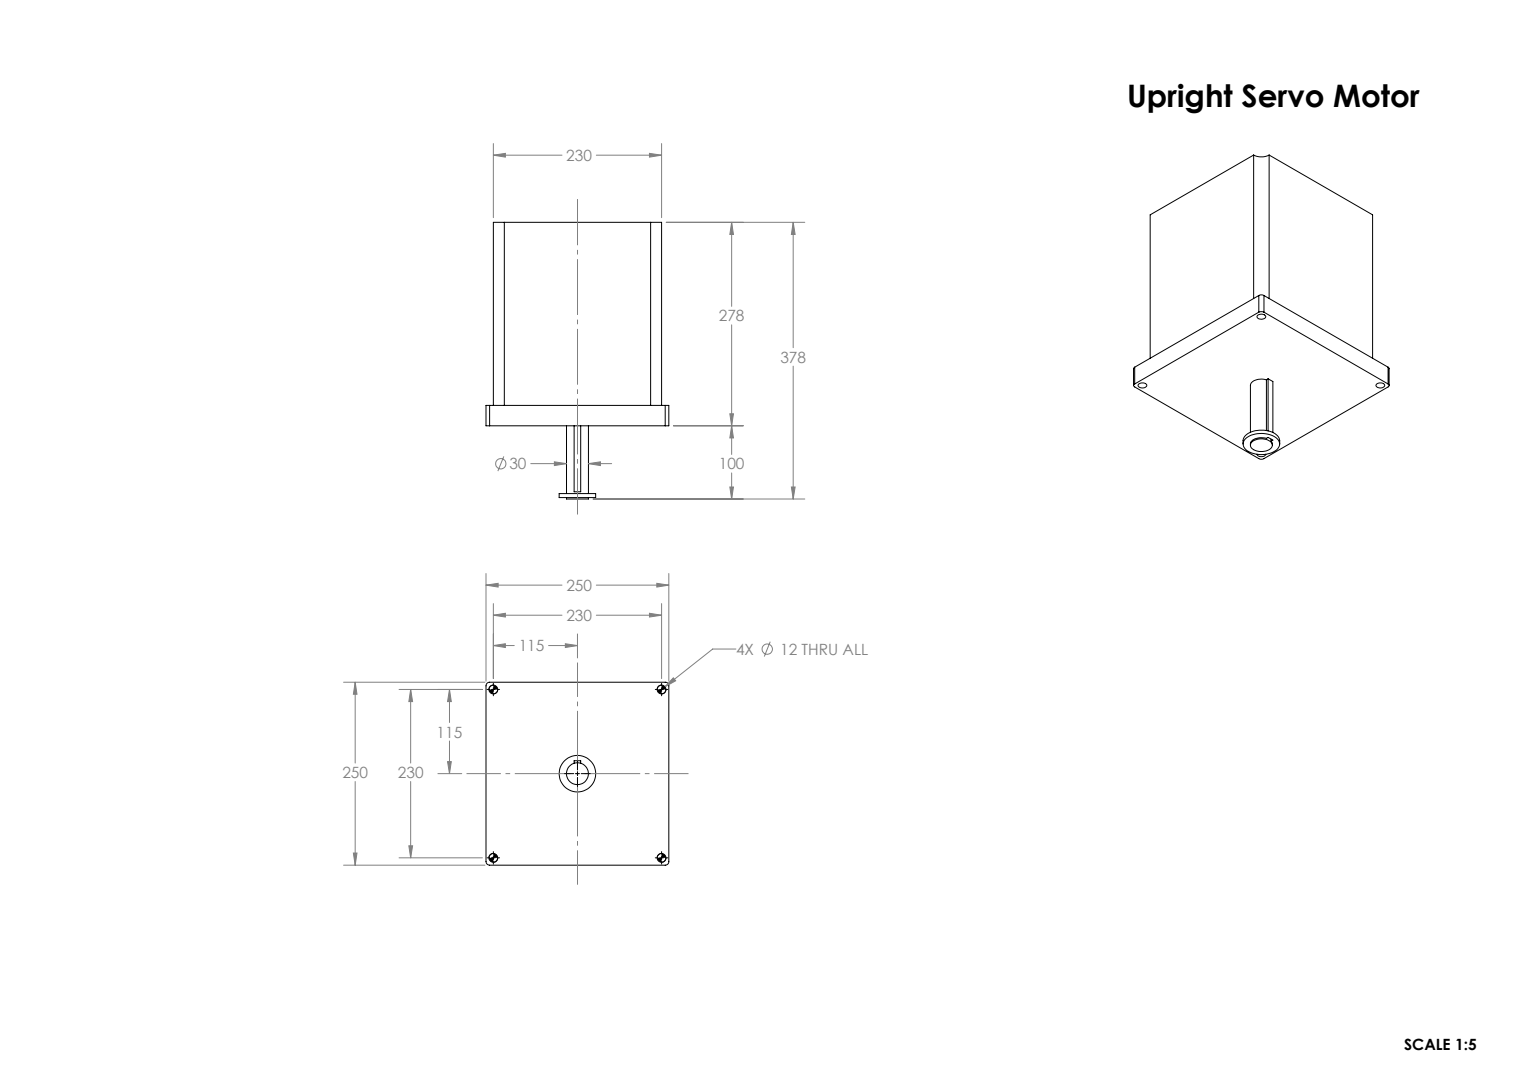
ISO-10303-21;
HEADER;
FILE_DESCRIPTION (('STEP AP214'),
    '1' );
FILE_NAME ('Upright servo motor.step',
    '2026-10-28T15:55:38',
    ( '' ),
    ( '' ),
    'SwSTEP 2.0',
    'SolidWorks 2025',
    '' );
FILE_SCHEMA (( 'AUTOMOTIVE_DESIGN' ));
ENDSEC;

DATA;
#1=CARTESIAN_POINT ( 'NONE',  ( -125.0000000000000000, -125.0000000000000000, 0.000000000000000000 ) ) ;
#8=CARTESIAN_POINT ( 'NONE',  ( 120.9999999999999005, 115.0000000000000000, -28.00000000000002487 ) ) ;
#18=ORIENTED_EDGE ( 'NONE', *, *, #6588, .T. ) ;
#27=CARTESIAN_POINT ( 'NONE',  ( -120.0000000000000000, 125.0000000000000000, -28.00000000000002487 ) ) ;
#29=ORIENTED_EDGE ( 'NONE', *, *, #180, .F. ) ;
#40=ADVANCED_FACE ( 'NONE', ( #3535 ), #4054, .T. ) ;
#42=ADVANCED_FACE ( 'NONE', ( #6164, #8163 ), #4942, .F. ) ;
#56=LINE ( 'NONE', #2567, #4947 ) ;
#61=EDGE_LOOP ( 'NONE', ( #697, #3265, #3475, #7513, #3300, #8064, #2980, #925, #7599, #4514 ) ) ;
#65=CARTESIAN_POINT ( 'NONE',  ( 120.0000000000000000, 125.0000000000000000, -28.00000000000002487 ) ) ;
#70=DIRECTION ( 'NONE',  ( 0.000000000000000000, 0.000000000000000000, -1.000000000000000000 ) ) ;
#72=ADVANCED_FACE ( 'NONE', ( #4004 ), #7908, .T. ) ;
#79=AXIS2_PLACEMENT_3D ( 'NONE', #2314, #7459, #4304 ) ;
#83=DIRECTION ( 'NONE',  ( -0.000000000000000000, -1.000000000000000000, 0.000000000000000000 ) ) ;
#105=CIRCLE ( 'NONE', #5900, 5.000000000000004441 ) ;
#108=VECTOR ( 'NONE', #4963, 1000.000000000000000 ) ;
#116=ORIENTED_EDGE ( 'NONE', *, *, #2238, .T. ) ;
#122=DIRECTION ( 'NONE',  ( 0.000000000000000000, 0.000000000000000000, -1.000000000000000000 ) ) ;
#141=LINE ( 'NONE', #5340, #3208 ) ;
#159=CARTESIAN_POINT ( 'NONE',  ( -114.9999999999999147, 115.0000000000000000, 8.205133554287239938E-16 ) ) ;
#173=DIRECTION ( 'NONE',  ( -1.000000000000000000, 0.000000000000000000, 0.000000000000000000 ) ) ;
#175=AXIS2_PLACEMENT_3D ( 'NONE', #7870, #4041, #5363 ) ;
#177=ADVANCED_FACE ( 'NONE', ( #1614 ), #1876, .F. ) ;
#179=VERTEX_POINT ( 'NONE', #7618 ) ;
#180=EDGE_CURVE ( 'NONE', #860, #2097, #1404, .T. ) ;
#181=FACE_OUTER_BOUND ( 'NONE', #3614, .T. ) ;
#183=CARTESIAN_POINT ( 'NONE',  ( -15.00000000000000000, 1.836970198721029589E-15, -120.5000000000000284 ) ) ;
#185=VECTOR ( 'NONE', #4186, 1000.000000000000000 ) ;
#190=EDGE_CURVE ( 'NONE', #8098, #1436, #474, .T. ) ;
#196=DIRECTION ( 'NONE',  ( -1.000000000000000000, 0.000000000000000000, 0.000000000000000000 ) ) ;
#198=EDGE_CURVE ( 'NONE', #5389, #4917, #4249, .T. ) ;
#207=ORIENTED_EDGE ( 'NONE', *, *, #1868, .F. ) ;
#208=DIRECTION ( 'NONE',  ( -0.000000000000000000, 0.000000000000000000, 1.000000000000000000 ) ) ;
#217=CARTESIAN_POINT ( 'NONE',  ( 17.61817604250836311, 0.000000000000000000, -28.00000000000002487 ) ) ;
#229=VECTOR ( 'NONE', #850, 1000.000000000000000 ) ;
#232=ORIENTED_EDGE ( 'NONE', *, *, #4651, .F. ) ;
#243=CIRCLE ( 'NONE', #6316, 15.00000000000001421 ) ;
#244=CIRCLE ( 'NONE', #3336, 5.999999999999991118 ) ;
#254=ORIENTED_EDGE ( 'NONE', *, *, #2828, .T. ) ;
#261=DIRECTION ( 'NONE',  ( -0.000000000000000000, -0.000000000000000000, -1.000000000000000000 ) ) ;
#271=CARTESIAN_POINT ( 'NONE',  ( 0.000000000000000000, -4.500000000000000000, -118.0000000000000284 ) ) ;
#286=EDGE_CURVE ( 'NONE', #441, #1522, #6503, .T. ) ;
#295=EDGE_CURVE ( 'NONE', #2535, #179, #3684, .T. ) ;
#300=CARTESIAN_POINT ( 'NONE',  ( -114.9999999999999147, 115.0000000000000000, 0.000000000000000000 ) ) ;
#304=DIRECTION ( 'NONE',  ( -0.000000000000000000, -0.000000000000000000, 1.000000000000000000 ) ) ;
#306=VERTEX_POINT ( 'NONE', #4470 ) ;
#308=EDGE_CURVE ( 'NONE', #902, #5541, #1677, .T. ) ;
#310=CLOSED_SHELL ( 'NONE', ( #3649, #1499, #7471, #6289, #6383, #2621, #654, #8259, #5840, #40, #7066, #4000, #7991, #7178, #2940, #72, #5941, #5722, #5455, #6114, #6194, #3420, #920, #177, #2590, #2030, #4073, #5503, #4001, #3296, #1919, #610, #4469, #5040, #3468, #42, #666, #5099, #4929, #6667, #3666 ) ) ;
#315=CARTESIAN_POINT ( 'NONE',  ( 0.000000000000000000, 0.000000000000000000, -128.0000000000000284 ) ) ;
#326=VERTEX_POINT ( 'NONE', #1488 ) ;
#331=LINE ( 'NONE', #1063, #1617 ) ;
#342=( NAMED_UNIT ( * ) SI_UNIT ( $, .STERADIAN. ) SOLID_ANGLE_UNIT ( ) );
#347=DIRECTION ( 'NONE',  ( -1.000000000000000000, 0.000000000000000000, -0.000000000000000000 ) ) ;
#350=AXIS2_PLACEMENT_3D ( 'NONE', #7544, #3683, #6944 ) ;
#352=DIRECTION ( 'NONE',  ( 1.000000000000000000, 0.000000000000000000, 0.000000000000000000 ) ) ;
#370=CARTESIAN_POINT ( 'NONE',  ( 0.000000000000000000, 0.000000000000000000, -120.5000000000000284 ) ) ;
#371=AXIS2_PLACEMENT_3D ( 'NONE', #2070, #6035, #7190 ) ;
#377=AXIS2_PLACEMENT_3D ( 'NONE', #5650, #8275, #3063 ) ;
#380=DIRECTION ( 'NONE',  ( -1.000000000000000000, 0.000000000000000000, 0.000000000000000000 ) ) ;
#381=VERTEX_POINT ( 'NONE', #27 ) ;
#383=AXIS2_PLACEMENT_3D ( 'NONE', #486, #7032, #3735 ) ;
#407=ORIENTED_EDGE ( 'NONE', *, *, #3693, .F. ) ;
#411=LINE ( 'NONE', #3703, #3911 ) ;
#415=FACE_OUTER_BOUND ( 'NONE', #707, .T. ) ;
#428=LINE ( 'NONE', #8161, #3975 ) ;
#430=CARTESIAN_POINT ( 'NONE',  ( 114.9999999999999147, 115.0000000000000000, 0.000000000000000000 ) ) ;
#433=EDGE_LOOP ( 'NONE', ( #2336, #6110, #4542, #3751 ) ) ;
#441=VERTEX_POINT ( 'NONE', #3239 ) ;
#450=DIRECTION ( 'NONE',  ( -1.000000000000000000, 0.000000000000000000, 0.000000000000000000 ) ) ;
#455=PLANE ( 'NONE',  #2955 ) ;
#465=CARTESIAN_POINT ( 'NONE',  ( -120.0000000000000000, -125.0000000000000000, 0.000000000000000000 ) ) ;
#471=VERTEX_POINT ( 'NONE', #3527 ) ;
#474=LINE ( 'NONE', #5587, #3002 ) ;
#475=FACE_OUTER_BOUND ( 'NONE', #6736, .T. ) ;
#486=CARTESIAN_POINT ( 'NONE',  ( -114.9999999999999147, -115.0000000000000000, 250.0000000000000000 ) ) ;
#493=DIRECTION ( 'NONE',  ( -0.000000000000000000, -0.000000000000000000, 1.000000000000000000 ) ) ;
#506=CARTESIAN_POINT ( 'NONE',  ( 17.61817604250836311, 0.000000000000000000, -128.0000120000000265 ) ) ;
#515=ORIENTED_EDGE ( 'NONE', *, *, #1831, .T. ) ;
#534=CIRCLE ( 'NONE', #1490, 5.000000000000004441 ) ;
#535=CARTESIAN_POINT ( 'NONE',  ( 0.000000000000000000, 0.000000000000000000, -128.0000000000000284 ) ) ;
#536=AXIS2_PLACEMENT_3D ( 'NONE', #6714, #5911, #8024 ) ;
#538=FACE_OUTER_BOUND ( 'NONE', #2255, .T. ) ;
#546=ORIENTED_EDGE ( 'NONE', *, *, #4676, .T. ) ;
#548=CARTESIAN_POINT ( 'NONE',  ( -125.0000000000000000, 125.0000000000000000, -28.00000000000002487 ) ) ;
#552=ORIENTED_EDGE ( 'NONE', *, *, #875, .F. ) ;
#559=ORIENTED_EDGE ( 'NONE', *, *, #4204, .F. ) ;
#565=DIRECTION ( 'NONE',  ( -1.000000000000000000, 0.000000000000000000, -0.000000000000000000 ) ) ;
#566=DIRECTION ( 'NONE',  ( -0.000000000000000000, -0.000000000000000000, 1.000000000000000000 ) ) ;
#570=EDGE_CURVE ( 'NONE', #6321, #3267, #1593, .T. ) ;
#578=FACE_OUTER_BOUND ( 'NONE', #61, .T. ) ;
#581=EDGE_CURVE ( 'NONE', #7933, #4405, #6106, .T. ) ;
#583=AXIS2_PLACEMENT_3D ( 'NONE', #4746, #5934, #7328 ) ;
#589=LINE ( 'NONE', #629, #1204 ) ;
#593=EDGE_LOOP ( 'NONE', ( #552, #7812 ) ) ;
#607=CIRCLE ( 'NONE', #7489, 5.999999999999991118 ) ;
#610=ADVANCED_FACE ( 'NONE', ( #5041 ), #4306, .T. ) ;
#612=EDGE_LOOP ( 'NONE', ( #6446, #1124, #2582, #4474, #7041 ) ) ;
#615=EDGE_CURVE ( 'NONE', #4158, #3739, #1807, .T. ) ;
#620=DIRECTION ( 'NONE',  ( 1.000000000000000000, -0.000000000000000000, 0.000000000000000000 ) ) ;
#629=CARTESIAN_POINT ( 'NONE',  ( -120.0000000000000000, -125.0000000000000000, -28.00000000000002487 ) ) ;
#633=VECTOR ( 'NONE', #208, 1000.000000000000000 ) ;
#644=LINE ( 'NONE', #2550, #3740 ) ;
#645=CARTESIAN_POINT ( 'NONE',  ( 114.9999999999999147, 115.0000000000000000, 250.0000000000000000 ) ) ;
#654=ADVANCED_FACE ( 'NONE', ( #5169 ), #7069, .F. ) ;
#659=DIRECTION ( 'NONE',  ( -1.000000000000000000, 0.000000000000000000, 0.000000000000000000 ) ) ;
#666=ADVANCED_FACE ( 'NONE', ( #5376 ), #6607, .T. ) ;
#668=ORIENTED_EDGE ( 'NONE', *, *, #4872, .F. ) ;
#672=EDGE_LOOP ( 'NONE', ( #3276, #4594, #7730, #8070 ) ) ;
#687=ORIENTED_EDGE ( 'NONE', *, *, #3635, .T. ) ;
#697=ORIENTED_EDGE ( 'NONE', *, *, #8210, .F. ) ;
#698=VERTEX_POINT ( 'NONE', #4611 ) ;
#703=LINE ( 'NONE', #5265, #4111 ) ;
#705=EDGE_LOOP ( 'NONE', ( #4300, #4268, #4984, #5088 ) ) ;
#706=MANIFOLD_SOLID_BREP ( 'Cut-Extrude1', #310 ) ;
#707=EDGE_LOOP ( 'NONE', ( #6265, #1176, #18, #8160, #1408, #795, #3196, #6738 ) ) ;
#720=CARTESIAN_POINT ( 'NONE',  ( 17.61817604250836311, 0.000000000000000000, -118.0000000000000284 ) ) ;
#733=DIRECTION ( 'NONE',  ( 0.000000000000000000, 0.000000000000000000, -1.000000000000000000 ) ) ;
#735=EDGE_CURVE ( 'NONE', #3015, #3602, #6056, .T. ) ;
#740=EDGE_CURVE ( 'NONE', #2575, #6246, #8045, .T. ) ;
#741=LINE ( 'NONE', #2603, #1864 ) ;
#744=LINE ( 'NONE', #906, #4238 ) ;
#748=ORIENTED_EDGE ( 'NONE', *, *, #2964, .F. ) ;
#751=CARTESIAN_POINT ( 'NONE',  ( -15.00000000000000000, 1.836970198721029589E-15, -128.0000000000000284 ) ) ;
#753=AXIS2_PLACEMENT_3D ( 'NONE', #5334, #785, #7918 ) ;
#755=EDGE_LOOP ( 'NONE', ( #6173, #4215, #4913, #5960 ) ) ;
#763=DIRECTION ( 'NONE',  ( -1.000000000000000000, 0.000000000000000000, 0.000000000000000000 ) ) ;
#766=LINE ( 'NONE', #1, #7092 ) ;
#776=PLANE ( 'NONE',  #6139 ) ;
#785=DIRECTION ( 'NONE',  ( 0.000000000000000000, 0.000000000000000000, 1.000000000000000000 ) ) ;
#786=CARTESIAN_POINT ( 'NONE',  ( 114.9999999999999147, 115.0000000000000000, 8.205133554287239938E-16 ) ) ;
#789=ORIENTED_EDGE ( 'NONE', *, *, #1988, .T. ) ;
#795=ORIENTED_EDGE ( 'NONE', *, *, #6434, .F. ) ;
#797=DIRECTION ( 'NONE',  ( 1.000000000000000000, 0.000000000000000000, 0.000000000000000000 ) ) ;
#802=CIRCLE ( 'NONE', #2559, 15.00000000000000178 ) ;
#805=VERTEX_POINT ( 'NONE', #4712 ) ;
#823=CARTESIAN_POINT ( 'NONE',  ( 0.000000000000000000, 0.000000000000000000, -128.0000000000000284 ) ) ;
#827=CARTESIAN_POINT ( 'NONE',  ( -15.00000000000000000, 1.836970198721029589E-15, -126.0000000000000284 ) ) ;
#831=DIRECTION ( 'NONE',  ( 1.000000000000000000, 0.000000000000000000, 0.000000000000000000 ) ) ;
#838=CARTESIAN_POINT ( 'NONE',  ( 0.000000000000000000, 4.500000000000000000, -126.0000000000000284 ) ) ;
#850=DIRECTION ( 'NONE',  ( -0.000000000000000000, -0.000000000000000000, 1.000000000000000000 ) ) ;
#857=CARTESIAN_POINT ( 'NONE',  ( 17.61817604250836311, 0.000000000000000000, -126.0000000000000284 ) ) ;
#859=EDGE_LOOP ( 'NONE', ( #1022, #5933, #4897, #7019 ) ) ;
#860=VERTEX_POINT ( 'NONE', #1420 ) ;
#869=DIRECTION ( 'NONE',  ( 1.000000000000000000, 0.000000000000000000, 0.000000000000000000 ) ) ;
#872=DIRECTION ( 'NONE',  ( -1.000000000000000000, 0.000000000000000000, 0.000000000000000000 ) ) ;
#875=EDGE_CURVE ( 'NONE', #5541, #902, #607, .T. ) ;
#897=CIRCLE ( 'NONE', #5065, 15.00000000000000000 ) ;
#900=VERTEX_POINT ( 'NONE', #1546 ) ;
#901=CIRCLE ( 'NONE', #2392, 5.999999999999991118 ) ;
#902=VERTEX_POINT ( 'NONE', #2874 ) ;
#906=CARTESIAN_POINT ( 'NONE',  ( -0.000000000000000000, -115.0000000000000000, 0.000000000000000000 ) ) ;
#911=VECTOR ( 'NONE', #1701, 1000.000000000000000 ) ;
#913=CIRCLE ( 'NONE', #5356, 15.00000000000000000 ) ;
#920=ADVANCED_FACE ( 'NONE', ( #4178 ), #7961, .T. ) ;
#925=ORIENTED_EDGE ( 'NONE', *, *, #2471, .F. ) ;
#926=CARTESIAN_POINT ( 'NONE',  ( -125.0000000000000000, -120.0000000000000000, 0.000000000000000000 ) ) ;
#934=CARTESIAN_POINT ( 'NONE',  ( -15.00000000000000000, 1.836970198721029589E-15, -128.0000000000000284 ) ) ;
#959=CARTESIAN_POINT ( 'NONE',  ( 125.0000000000000000, -120.0000000000000000, 0.000000000000000000 ) ) ;
#960=ORIENTED_EDGE ( 'NONE', *, *, #2835, .F. ) ;
#973=EDGE_CURVE ( 'NONE', #860, #2535, #428, .T. ) ;
#974=DIRECTION ( 'NONE',  ( -1.000000000000000000, 0.000000000000000000, 0.000000000000000000 ) ) ;
#991=EDGE_CURVE ( 'NONE', #1826, #2040, #4912, .T. ) ;
#998=DIRECTION ( 'NONE',  ( -0.000000000000000000, -0.000000000000000000, 1.000000000000000000 ) ) ;
#1006=VECTOR ( 'NONE', #4028, 1000.000000000000000 ) ;
#1010=VERTEX_POINT ( 'NONE', #7054 ) ;
#1011=DIRECTION ( 'NONE',  ( 1.000000000000000000, 0.000000000000000000, 0.000000000000000000 ) ) ;
#1013=EDGE_LOOP ( 'NONE', ( #559, #6984, #2873, #7573 ) ) ;
#1018=ORIENTED_EDGE ( 'NONE', *, *, #3827, .T. ) ;
#1022=ORIENTED_EDGE ( 'NONE', *, *, #5036, .F. ) ;
#1026=EDGE_CURVE ( 'NONE', #4868, #3146, #766, .T. ) ;
#1036=FACE_BOUND ( 'NONE', #3299, .T. ) ;
#1039=CIRCLE ( 'NONE', #8188, 15.00000000000000000 ) ;
#1040=CARTESIAN_POINT ( 'NONE',  ( 120.9999999999999005, 115.0000000000000000, 0.000000000000000000 ) ) ;
#1046=EDGE_CURVE ( 'NONE', #1156, #5510, #1993, .T. ) ;
#1052=DIRECTION ( 'NONE',  ( 0.000000000000000000, 0.000000000000000000, -1.000000000000000000 ) ) ;
#1055=ORIENTED_EDGE ( 'NONE', *, *, #2141, .T. ) ;
#1056=CIRCLE ( 'NONE', #2670, 14.99999999999998579 ) ;
#1057=ORIENTED_EDGE ( 'NONE', *, *, #4872, .T. ) ;
#1063=CARTESIAN_POINT ( 'NONE',  ( 114.9999999999999147, -100.0000000000000000, 250.0000000000000000 ) ) ;
#1092=CARTESIAN_POINT ( 'NONE',  ( 114.9999999999999147, 99.99999999999998579, 250.0000000000000000 ) ) ;
#1100=EDGE_LOOP ( 'NONE', ( #2705, #116, #7783, #4128 ) ) ;
#1104=LINE ( 'NONE', #3664, #3805 ) ;
#1108=ORIENTED_EDGE ( 'NONE', *, *, #1831, .F. ) ;
#1114=ORIENTED_EDGE ( 'NONE', *, *, #740, .F. ) ;
#1116=DIRECTION ( 'NONE',  ( -0.000000000000000000, -0.000000000000000000, -1.000000000000000000 ) ) ;
#1124=ORIENTED_EDGE ( 'NONE', *, *, #6601, .F. ) ;
#1128=FACE_BOUND ( 'NONE', #2832, .T. ) ;
#1135=EDGE_CURVE ( 'NONE', #5480, #5616, #901, .T. ) ;
#1139=LINE ( 'NONE', #6232, #5220 ) ;
#1151=CARTESIAN_POINT ( 'NONE',  ( 120.0000000000000000, 120.0000000000000000, 0.000000000000000000 ) ) ;
#1153=ORIENTED_EDGE ( 'NONE', *, *, #2768, .T. ) ;
#1156=VERTEX_POINT ( 'NONE', #7787 ) ;
#1170=DIRECTION ( 'NONE',  ( 0.000000000000000000, -0.000000000000000000, -1.000000000000000000 ) ) ;
#1174=DIRECTION ( 'NONE',  ( -0.000000000000000000, -0.000000000000000000, -1.000000000000000000 ) ) ;
#1176=ORIENTED_EDGE ( 'NONE', *, *, #7255, .T. ) ;
#1178=ORIENTED_EDGE ( 'NONE', *, *, #7163, .F. ) ;
#1193=EDGE_LOOP ( 'NONE', ( #3836, #2902 ) ) ;
#1196=CARTESIAN_POINT ( 'NONE',  ( 114.9999999999999147, -100.0000000000000000, 250.0000000000000000 ) ) ;
#1204=VECTOR ( 'NONE', #7735, 1000.000000000000000 ) ;
#1215=LINE ( 'NONE', #3138, #8195 ) ;
#1220=ORIENTED_EDGE ( 'NONE', *, *, #740, .T. ) ;
#1223=ORIENTED_EDGE ( 'NONE', *, *, #8210, .T. ) ;
#1224=DIRECTION ( 'NONE',  ( -0.000000000000000000, -0.000000000000000000, 1.000000000000000000 ) ) ;
#1230=ORIENTED_EDGE ( 'NONE', *, *, #5274, .T. ) ;
#1236=LINE ( 'NONE', #5104, #2277 ) ;
#1242=CARTESIAN_POINT ( 'NONE',  ( -114.9999999999999147, -115.0000000000000000, -28.00000000000002487 ) ) ;
#1246=DIRECTION ( 'NONE',  ( 1.000000000000000000, 0.000000000000000000, 0.000000000000000000 ) ) ;
#1258=PLANE ( 'NONE',  #5615 ) ;
#1259=AXIS2_PLACEMENT_3D ( 'NONE', #645, #5115, #2551 ) ;
#1264=DIRECTION ( 'NONE',  ( 1.000000000000000000, 0.000000000000000000, 0.000000000000000000 ) ) ;
#1273=EDGE_CURVE ( 'NONE', #2993, #326, #2375, .T. ) ;
#1278=DIRECTION ( 'NONE',  ( -0.000000000000000000, -0.000000000000000000, 1.000000000000000000 ) ) ;
#1285=EDGE_CURVE ( 'NONE', #2048, #805, #1104, .T. ) ;
#1291=FACE_OUTER_BOUND ( 'NONE', #6963, .T. ) ;
#1298=FACE_OUTER_BOUND ( 'NONE', #2580, .T. ) ;
#1299=AXIS2_PLACEMENT_3D ( 'NONE', #5884, #1507, #5927 ) ;
#1315=CIRCLE ( 'NONE', #79, 5.999999999999991118 ) ;
#1322=VECTOR ( 'NONE', #6685, 1000.000000000000000 ) ;
#1332=CARTESIAN_POINT ( 'NONE',  ( 108.9999999999999147, 115.0000000000000000, 8.205133554287239938E-16 ) ) ;
#1338=AXIS2_PLACEMENT_3D ( 'NONE', #7250, #6573, #797 ) ;
#1352=AXIS2_PLACEMENT_3D ( 'NONE', #2473, #566, #6940 ) ;
#1364=DIRECTION ( 'NONE',  ( -1.000000000000000000, 0.000000000000000000, 0.000000000000000000 ) ) ;
#1373=DIRECTION ( 'NONE',  ( -1.000000000000000000, 0.000000000000000000, 0.000000000000000000 ) ) ;
#1402=VERTEX_POINT ( 'NONE', #5132 ) ;
#1403=DIRECTION ( 'NONE',  ( 0.000000000000000000, 0.000000000000000000, 1.000000000000000000 ) ) ;
#1404=CIRCLE ( 'NONE', #2867, 5.999999999999991118 ) ;
#1408=ORIENTED_EDGE ( 'NONE', *, *, #7184, .F. ) ;
#1420=CARTESIAN_POINT ( 'NONE',  ( -120.9999999999999005, 115.0000000000000000, -28.00000000000002487 ) ) ;
#1436=VERTEX_POINT ( 'NONE', #2152 ) ;
#1439=EDGE_CURVE ( 'NONE', #3146, #2918, #7043, .T. ) ;
#1440=SHAPE_REPRESENTATION ( 'Upright servo motor', ( #1299 ), #7463 ) ;
#1446=VECTOR ( 'NONE', #1666, 1000.000000000000000 ) ;
#1457=CIRCLE ( 'NONE', #3320, 25.00000000000000000 ) ;
#1465=AXIS2_PLACEMENT_3D ( 'NONE', #1830, #7610, #3840 ) ;
#1468=ORIENTED_EDGE ( 'NONE', *, *, #7255, .F. ) ;
#1474=LINE ( 'NONE', #6445, #5413 ) ;
#1479=CARTESIAN_POINT ( 'NONE',  ( 108.9999999999999147, 115.0000000000000000, -28.00000000000002487 ) ) ;
#1488=CARTESIAN_POINT ( 'NONE',  ( -114.9999999999999147, 99.99999999999998579, 0.000000000000000000 ) ) ;
#1490=AXIS2_PLACEMENT_3D ( 'NONE', #6464, #733, #6414 ) ;
#1499=ADVANCED_FACE ( 'NONE', ( #6568 ), #3346, .F. ) ;
#1504=CARTESIAN_POINT ( 'NONE',  ( 0.000000000000000000, 0.000000000000000000, -118.0000000000000284 ) ) ;
#1507=DIRECTION ( 'NONE',  ( 0.000000000000000000, 0.000000000000000000, 1.000000000000000000 ) ) ;
#1510=ORIENTED_EDGE ( 'NONE', *, *, #2685, .F. ) ;
#1513=CARTESIAN_POINT ( 'NONE',  ( 114.9999999999999147, 115.0000000000000000, 250.0000000000000000 ) ) ;
#1521=CARTESIAN_POINT ( 'NONE',  ( 0.000000000000000000, 0.000000000000000000, -118.0000000000000284 ) ) ;
#1522=VERTEX_POINT ( 'NONE', #6085 ) ;
#1531=CYLINDRICAL_SURFACE ( 'NONE', #1465, 5.000000000000004441 ) ;
#1546=CARTESIAN_POINT ( 'NONE',  ( 108.9999999999999147, -115.0000000000000000, 8.205133554287239938E-16 ) ) ;
#1550=AXIS2_PLACEMENT_3D ( 'NONE', #7363, #4133, #173 ) ;
#1554=DIRECTION ( 'NONE',  ( -0.000000000000000000, -0.000000000000000000, 1.000000000000000000 ) ) ;
#1558=( NAMED_UNIT ( * ) PLANE_ANGLE_UNIT ( ) SI_UNIT ( $, .RADIAN. ) );
#1563=CARTESIAN_POINT ( 'NONE',  ( 0.000000000000000000, -115.0000000000000000, 250.0000000000000000 ) ) ;
#1573=PLANE ( 'NONE',  #536 ) ;
#1587=DIRECTION ( 'NONE',  ( 0.000000000000000000, 1.000000000000000000, 0.000000000000000000 ) ) ;
#1593=LINE ( 'NONE', #4103, #1006 ) ;
#1602=ORIENTED_EDGE ( 'NONE', *, *, #1646, .T. ) ;
#1606=ORIENTED_EDGE ( 'NONE', *, *, #3419, .F. ) ;
#1607=CARTESIAN_POINT ( 'NONE',  ( 0.000000000000000000, 0.000000000000000000, -28.00000000000002487 ) ) ;
#1610=CARTESIAN_POINT ( 'NONE',  ( -108.9999999999999147, 115.0000000000000000, -28.00000000000002487 ) ) ;
#1612=DIRECTION ( 'NONE',  ( -1.000000000000000000, 0.000000000000000000, 0.000000000000000000 ) ) ;
#1614=FACE_OUTER_BOUND ( 'NONE', #3031, .T. ) ;
#1617=VECTOR ( 'NONE', #3669, 1000.000000000000000 ) ;
#1618=VERTEX_POINT ( 'NONE', #2962 ) ;
#1642=CARTESIAN_POINT ( 'NONE',  ( 0.000000000000000000, 4.500000000000000000, -28.00000000000002487 ) ) ;
#1646=EDGE_CURVE ( 'NONE', #3602, #4182, #8060, .T. ) ;
#1659=CARTESIAN_POINT ( 'NONE',  ( -99.99999999999990052, 115.0000000000000000, 250.0000000000000000 ) ) ;
#1666=DIRECTION ( 'NONE',  ( -0.000000000000000000, -0.000000000000000000, -1.000000000000000000 ) ) ;
#1677=CIRCLE ( 'NONE', #8291, 5.999999999999991118 ) ;
#1680=VERTEX_POINT ( 'NONE', #4849 ) ;
#1701=DIRECTION ( 'NONE',  ( -0.000000000000000000, -0.000000000000000000, -1.000000000000000000 ) ) ;
#1712=PLANE ( 'NONE',  #6288 ) ;
#1714=ORIENTED_EDGE ( 'NONE', *, *, #3909, .F. ) ;
#1720=AXIS2_PLACEMENT_3D ( 'NONE', #4653, #6681, #4610 ) ;
#1725=DIRECTION ( 'NONE',  ( 0.000000000000000000, 0.000000000000000000, 1.000000000000000000 ) ) ;
#1728=EDGE_LOOP ( 'NONE', ( #232, #5693, #3645, #5839 ) ) ;
#1739=DIRECTION ( 'NONE',  ( -0.000000000000000000, -0.000000000000000000, 1.000000000000000000 ) ) ;
#1745=EDGE_CURVE ( 'NONE', #7187, #2575, #4891, .T. ) ;
#1764=FACE_BOUND ( 'NONE', #612, .T. ) ;
#1767=DIRECTION ( 'NONE',  ( -1.000000000000000000, 0.000000000000000000, 0.000000000000000000 ) ) ;
#1776=ORIENTED_EDGE ( 'NONE', *, *, #4676, .F. ) ;
#1787=VERTEX_POINT ( 'NONE', #3399 ) ;
#1788=ORIENTED_EDGE ( 'NONE', *, *, #1439, .T. ) ;
#1794=LINE ( 'NONE', #3627, #6152 ) ;
#1795=AXIS2_PLACEMENT_3D ( 'NONE', #3418, #3382, #872 ) ;
#1807=LINE ( 'NONE', #1040, #8016 ) ;
#1808=CARTESIAN_POINT ( 'NONE',  ( 0.000000000000000000, 115.0000000000000000, 250.0000000000000000 ) ) ;
#1814=AXIS2_PLACEMENT_3D ( 'NONE', #3162, #8332, #5070 ) ;
#1818=CARTESIAN_POINT ( 'NONE',  ( -120.9999999999999005, -115.0000000000000000, -28.00000000000002487 ) ) ;
#1826=VERTEX_POINT ( 'NONE', #2707 ) ;
#1828=MECHANICAL_DESIGN_GEOMETRIC_PRESENTATION_REPRESENTATION('',(#3014),#4768);
#1830=CARTESIAN_POINT ( 'NONE',  ( -120.0000000000000000, 120.0000000000000000, -28.00000000000002487 ) ) ;
#1831=EDGE_CURVE ( 'NONE', #900, #7564, #7396, .T. ) ;
#1843=CYLINDRICAL_SURFACE ( 'NONE', #2399, 5.999999999999991118 ) ;
#1845=LINE ( 'NONE', #8344, #3612 ) ;
#1855=UNCERTAINTY_MEASURE_WITH_UNIT (LENGTH_MEASURE( 1.000000000000000082E-05 ), #3540, 'distance_accuracy_value', 'NONE');
#1856=ORIENTED_EDGE ( 'NONE', *, *, #6275, .T. ) ;
#1859=EDGE_LOOP ( 'NONE', ( #789, #2881, #5851, #4229, #5350 ) ) ;
#1860=CARTESIAN_POINT ( 'NONE',  ( 0.000000000000000000, 4.500000000000000000, -118.0000000000000284 ) ) ;
#1864=VECTOR ( 'NONE', #5763, 1000.000000000000000 ) ;
#1868=EDGE_CURVE ( 'NONE', #5616, #5480, #4408, .T. ) ;
#1876=CYLINDRICAL_SURFACE ( 'NONE', #1814, 15.00000000000000000 ) ;
#1886=CARTESIAN_POINT ( 'NONE',  ( 0.000000000000000000, 0.000000000000000000, -126.0000000000000284 ) ) ;
#1891=ORIENTED_EDGE ( 'NONE', *, *, #7608, .F. ) ;
#1919=ADVANCED_FACE ( 'NONE', ( #2008 ), #5194, .T. ) ;
#1920=DIRECTION ( 'NONE',  ( 1.000000000000000000, 0.000000000000000000, 0.000000000000000000 ) ) ;
#1925=CARTESIAN_POINT ( 'NONE',  ( 17.61817604250836311, 4.500000000000000000, -120.5000000000000284 ) ) ;
#1928=DIRECTION ( 'NONE',  ( 1.000000000000000000, 0.000000000000000000, 0.000000000000000000 ) ) ;
#1937=DIRECTION ( 'NONE',  ( 0.000000000000000000, 1.000000000000000000, 0.000000000000000000 ) ) ;
#1938=EDGE_CURVE ( 'NONE', #5315, #1010, #2286, .T. ) ;
#1939=LINE ( 'NONE', #1808, #6729 ) ;
#1962=VERTEX_POINT ( 'NONE', #3358 ) ;
#1963=ORIENTED_EDGE ( 'NONE', *, *, #4837, .F. ) ;
#1978=ORIENTED_EDGE ( 'NONE', *, *, #1026, .F. ) ;
#1988=EDGE_CURVE ( 'NONE', #1680, #6868, #7261, .T. ) ;
#1990=EDGE_CURVE ( 'NONE', #4182, #4386, #8216, .T. ) ;
#1992=ORIENTED_EDGE ( 'NONE', *, *, #5607, .F. ) ;
#1993=CIRCLE ( 'NONE', #3040, 25.00000000000000000 ) ;
#2008=FACE_OUTER_BOUND ( 'NONE', #8041, .T. ) ;
#2016=DIRECTION ( 'NONE',  ( 1.000000000000000000, 0.000000000000000000, 0.000000000000000000 ) ) ;
#2019=VERTEX_POINT ( 'NONE', #3396 ) ;
#2029=FACE_OUTER_BOUND ( 'NONE', #6543, .T. ) ;
#2030=ADVANCED_FACE ( 'NONE', ( #415 ), #8104, .T. ) ;
#2040=VERTEX_POINT ( 'NONE', #8147 ) ;
#2044=VECTOR ( 'NONE', #3445, 1000.000000000000000 ) ;
#2048=VERTEX_POINT ( 'NONE', #6067 ) ;
#2050=VECTOR ( 'NONE', #7364, 1000.000000000000000 ) ;
#2055=DIRECTION ( 'NONE',  ( -1.000000000000000000, 0.000000000000000000, 0.000000000000000000 ) ) ;
#2058=DIRECTION ( 'NONE',  ( -0.000000000000000000, -0.000000000000000000, -1.000000000000000000 ) ) ;
#2070=CARTESIAN_POINT ( 'NONE',  ( 114.9999999999999147, -115.0000000000000000, 8.205133554287239938E-16 ) ) ;
#2097=VERTEX_POINT ( 'NONE', #1610 ) ;
#2098=AXIS2_PLACEMENT_3D ( 'NONE', #4174, #6763, #5459 ) ;
#2102=DIRECTION ( 'NONE',  ( -0.000000000000000000, -0.000000000000000000, 1.000000000000000000 ) ) ;
#2104=LINE ( 'NONE', #5410, #2044 ) ;
#2108=CARTESIAN_POINT ( 'NONE',  ( 0.000000000000000000, 0.000000000000000000, -118.0000000000000284 ) ) ;
#2119=ORIENTED_EDGE ( 'NONE', *, *, #2298, .T. ) ;
#2132=CARTESIAN_POINT ( 'NONE',  ( 0.000000000000000000, 0.000000000000000000, -28.00000000000002487 ) ) ;
#2137=FACE_OUTER_BOUND ( 'NONE', #8280, .T. ) ;
#2140=CYLINDRICAL_SURFACE ( 'NONE', #5625, 25.00000000000000000 ) ;
#2141=EDGE_CURVE ( 'NONE', #4379, #1618, #7164, .T. ) ;
#2145=DIRECTION ( 'NONE',  ( 0.000000000000000000, 0.000000000000000000, -1.000000000000000000 ) ) ;
#2151=VECTOR ( 'NONE', #7134, 1000.000000000000000 ) ;
#2152=CARTESIAN_POINT ( 'NONE',  ( 120.0000000000000000, -125.0000000000000000, -28.00000000000002487 ) ) ;
#2169=AXIS2_PLACEMENT_3D ( 'NONE', #4286, #3713, #6244 ) ;
#2170=CARTESIAN_POINT ( 'NONE',  ( 120.0000000000000000, 120.0000000000000000, -28.00000000000002487 ) ) ;
#2192=CARTESIAN_POINT ( 'NONE',  ( 0.000000000000000000, -115.0000000000000000, 250.0000000000000000 ) ) ;
#2197=VECTOR ( 'NONE', #4070, 1000.000000000000000 ) ;
#2207=VECTOR ( 'NONE', #5535, 1000.000000000000000 ) ;
#2209=ORIENTED_EDGE ( 'NONE', *, *, #4753, .T. ) ;
#2210=DIRECTION ( 'NONE',  ( -1.000000000000000000, 0.000000000000000000, 0.000000000000000000 ) ) ;
#2233=DIRECTION ( 'NONE',  ( 1.000000000000000000, 0.000000000000000000, 0.000000000000000000 ) ) ;
#2238=EDGE_CURVE ( 'NONE', #698, #1826, #5980, .T. ) ;
#2240=CARTESIAN_POINT ( 'NONE',  ( -114.9999999999999147, -115.0000000000000000, 0.000000000000000000 ) ) ;
#2255=EDGE_LOOP ( 'NONE', ( #6356, #1114, #407, #3447 ) ) ;
#2261=DIRECTION ( 'NONE',  ( -0.000000000000000000, -0.000000000000000000, 1.000000000000000000 ) ) ;
#2273=VECTOR ( 'NONE', #1587, 1000.000000000000000 ) ;
#2277=VECTOR ( 'NONE', #6283, 1000.000000000000000 ) ;
#2283=FACE_OUTER_BOUND ( 'NONE', #2504, .T. ) ;
#2286=CIRCLE ( 'NONE', #7538, 25.00000000000000000 ) ;
#2289=VECTOR ( 'NONE', #5780, 1000.000000000000000 ) ;
#2291=VERTEX_POINT ( 'NONE', #5276 ) ;
#2292=CARTESIAN_POINT ( 'NONE',  ( -114.9999999999999147, 115.0000000000000000, 250.0000000000000000 ) ) ;
#2298=EDGE_CURVE ( 'NONE', #179, #2535, #3370, .T. ) ;
#2303=ORIENTED_EDGE ( 'NONE', *, *, #5622, .T. ) ;
#2308=DIRECTION ( 'NONE',  ( -0.000000000000000000, -0.000000000000000000, 1.000000000000000000 ) ) ;
#2314=CARTESIAN_POINT ( 'NONE',  ( 114.9999999999999147, -115.0000000000000000, -28.00000000000002487 ) ) ;
#2336=ORIENTED_EDGE ( 'NONE', *, *, #6917, .F. ) ;
#2354=DIRECTION ( 'NONE',  ( 0.000000000000000000, 0.000000000000000000, -1.000000000000000000 ) ) ;
#2355=AXIS2_PLACEMENT_3D ( 'NONE', #5502, #5073, #565 ) ;
#2362=DIRECTION ( 'NONE',  ( 1.000000000000000000, 0.000000000000000000, 0.000000000000000000 ) ) ;
#2364=LINE ( 'NONE', #1642, #2683 ) ;
#2369=CARTESIAN_POINT ( 'NONE',  ( 125.0000000000000000, 120.0000000000000000, 0.000000000000000000 ) ) ;
#2374=ORIENTED_EDGE ( 'NONE', *, *, #2964, .T. ) ;
#2375=LINE ( 'NONE', #6789, #2207 ) ;
#2377=LINE ( 'NONE', #5538, #4951 ) ;
#2379=EDGE_CURVE ( 'NONE', #1680, #7933, #1474, .T. ) ;
#2392=AXIS2_PLACEMENT_3D ( 'NONE', #1242, #7097, #6374 ) ;
#2396=FACE_BOUND ( 'NONE', #1193, .T. ) ;
#2399=AXIS2_PLACEMENT_3D ( 'NONE', #6177, #998, #3636 ) ;
#2403=EDGE_LOOP ( 'NONE', ( #7213, #1856, #1606, #4809, #4115, #6782, #5578, #1788 ) ) ;
#2412=FACE_OUTER_BOUND ( 'NONE', #6937, .T. ) ;
#2413=CARTESIAN_POINT ( 'NONE',  ( 17.61817604250836311, 4.500000000000000000, -28.00000000000002487 ) ) ;
#2422=CARTESIAN_POINT ( 'NONE',  ( 0.000000000000000000, 4.500000000000000000, -128.0000120000000265 ) ) ;
#2433=CIRCLE ( 'NONE', #4974, 25.00000000000000000 ) ;
#2440=AXIS2_PLACEMENT_3D ( 'NONE', #8286, #304, #1920 ) ;
#2445=ORIENTED_EDGE ( 'NONE', *, *, #5036, .T. ) ;
#2446=DIRECTION ( 'NONE',  ( 0.000000000000000000, -0.000000000000000000, -1.000000000000000000 ) ) ;
#2455=ORIENTED_EDGE ( 'NONE', *, *, #5475, .T. ) ;
#2464=DIRECTION ( 'NONE',  ( -1.000000000000000000, 0.000000000000000000, 0.000000000000000000 ) ) ;
#2467=CARTESIAN_POINT ( 'NONE',  ( 17.61817604250836311, -4.500000000000000000, -118.0000000000000284 ) ) ;
#2471=EDGE_CURVE ( 'NONE', #1962, #4206, #4109, .T. ) ;
#2473=CARTESIAN_POINT ( 'NONE',  ( 114.9999999999999147, 115.0000000000000000, -28.00000000000002487 ) ) ;
#2482=FACE_BOUND ( 'NONE', #3016, .T. ) ;
#2483=DIRECTION ( 'NONE',  ( -1.000000000000000000, 0.000000000000000000, 0.000000000000000000 ) ) ;
#2491=ORIENTED_EDGE ( 'NONE', *, *, #7743, .F. ) ;
#2504=EDGE_LOOP ( 'NONE', ( #2693, #207, #1057, #4728 ) ) ;
#2511=DIRECTION ( 'NONE',  ( 1.000000000000000000, 0.000000000000000000, 0.000000000000000000 ) ) ;
#2519=AXIS2_PLACEMENT_3D ( 'NONE', #6683, #3377, #2838 ) ;
#2531=ORIENTED_EDGE ( 'NONE', *, *, #3653, .F. ) ;
#2532=PRODUCT_DEFINITION_CONTEXT ( 'detailed design', #3212, 'design' ) ;
#2535=VERTEX_POINT ( 'NONE', #7971 ) ;
#2550=CARTESIAN_POINT ( 'NONE',  ( 114.9999999999999147, 0.000000000000000000, 0.000000000000000000 ) ) ;
#2551=DIRECTION ( 'NONE',  ( 1.000000000000000000, 0.000000000000000000, 0.000000000000000000 ) ) ;
#2557=ORIENTED_EDGE ( 'NONE', *, *, #3827, .F. ) ;
#2559=AXIS2_PLACEMENT_3D ( 'NONE', #1504, #2145, #3940 ) ;
#2560=AXIS2_PLACEMENT_3D ( 'NONE', #6311, #5200, #7545 ) ;
#2561=CARTESIAN_POINT ( 'NONE',  ( 14.30908802125418511, 4.500000000000000000, -28.00000000000002487 ) ) ;
#2562=CARTESIAN_POINT ( 'NONE',  ( -125.0000000000000000, 125.0000000000000000, -28.00000000000002487 ) ) ;
#2567=CARTESIAN_POINT ( 'NONE',  ( 120.0000000000000000, -125.0000000000000000, -28.00000000000002487 ) ) ;
#2568=ORIENTED_EDGE ( 'NONE', *, *, #3133, .T. ) ;
#2573=CARTESIAN_POINT ( 'NONE',  ( -25.00000000000000000, 0.000000000000000000, -128.0000000000000284 ) ) ;
#2575=VERTEX_POINT ( 'NONE', #1092 ) ;
#2580=EDGE_LOOP ( 'NONE', ( #8196, #4007, #1468, #8242 ) ) ;
#2582=ORIENTED_EDGE ( 'NONE', *, *, #1990, .F. ) ;
#2585=EDGE_CURVE ( 'NONE', #6321, #2993, #4961, .T. ) ;
#2590=ADVANCED_FACE ( 'NONE', ( #538 ), #8179, .F. ) ;
#2591=DIRECTION ( 'NONE',  ( -0.000000000000000000, -0.000000000000000000, -1.000000000000000000 ) ) ;
#2596=ORIENTED_EDGE ( 'NONE', *, *, #2379, .F. ) ;
#2603=CARTESIAN_POINT ( 'NONE',  ( 25.00000000000000000, 3.061616997868383043E-15, -128.0000000000000284 ) ) ;
#2613=ORIENTED_EDGE ( 'NONE', *, *, #7528, .F. ) ;
#2616=EDGE_CURVE ( 'NONE', #4104, #3739, #5336, .T. ) ;
#2620=VECTOR ( 'NONE', #1116, 1000.000000000000000 ) ;
#2621=ADVANCED_FACE ( 'NONE', ( #578 ), #7594, .T. ) ;
#2629=ORIENTED_EDGE ( 'NONE', *, *, #2379, .T. ) ;
#2633=DIRECTION ( 'NONE',  ( -0.000000000000000000, -0.000000000000000000, -1.000000000000000000 ) ) ;
#2639=ORIENTED_EDGE ( 'NONE', *, *, #5260, .T. ) ;
#2640=EDGE_CURVE ( 'NONE', #1680, #1522, #5005, .T. ) ;
#2646=DIRECTION ( 'NONE',  ( -0.000000000000000000, 0.000000000000000000, 1.000000000000000000 ) ) ;
#2651=ORIENTED_EDGE ( 'NONE', *, *, #6791, .F. ) ;
#2660=LINE ( 'NONE', #7974, #2151 ) ;
#2670=AXIS2_PLACEMENT_3D ( 'NONE', #7208, #5939, #4628 ) ;
#2675=FACE_OUTER_BOUND ( 'NONE', #4531, .T. ) ;
#2683=VECTOR ( 'NONE', #4190, 1000.000000000000000 ) ;
#2685=EDGE_CURVE ( 'NONE', #306, #7564, #6522, .T. ) ;
#2688=ORIENTED_EDGE ( 'NONE', *, *, #6794, .F. ) ;
#2693=ORIENTED_EDGE ( 'NONE', *, *, #6105, .F. ) ;
#2705=ORIENTED_EDGE ( 'NONE', *, *, #3419, .T. ) ;
#2706=CARTESIAN_POINT ( 'NONE',  ( -120.0000000000000000, -120.0000000000000000, 0.000000000000000000 ) ) ;
#2707=CARTESIAN_POINT ( 'NONE',  ( 120.0000000000000000, 125.0000000000000000, -28.00000000000002487 ) ) ;
#2711=DIRECTION ( 'NONE',  ( -1.000000000000000000, 0.000000000000000000, 0.000000000000000000 ) ) ;
#2726=ORIENTED_EDGE ( 'NONE', *, *, #3628, .F. ) ;
#2729=LINE ( 'NONE', #838, #3335 ) ;
#2743=PLANE ( 'NONE',  #6305 ) ;
#2746=DIRECTION ( 'NONE',  ( 0.000000000000000000, 1.000000000000000000, -0.000000000000000000 ) ) ;
#2753=FACE_OUTER_BOUND ( 'NONE', #2804, .T. ) ;
#2759=CYLINDRICAL_SURFACE ( 'NONE', #3605, 15.00000000000001421 ) ;
#2768=EDGE_CURVE ( 'NONE', #1436, #3146, #56, .T. ) ;
#2772=DIRECTION ( 'NONE',  ( 0.000000000000000000, -1.000000000000000000, 0.000000000000000000 ) ) ;
#2789=AXIS2_PLACEMENT_3D ( 'NONE', #2998, #4857, #3721 ) ;
#2790=AXIS2_PLACEMENT_3D ( 'NONE', #2132, #6541, #763 ) ;
#2797=CARTESIAN_POINT ( 'NONE',  ( 125.0000000000000000, 120.0000000000000000, 0.000000000000000000 ) ) ;
#2804=EDGE_LOOP ( 'NONE', ( #546, #6753 ) ) ;
#2805=CARTESIAN_POINT ( 'NONE',  ( -120.0000000000000000, 120.0000000000000000, 0.000000000000000000 ) ) ;
#2807=CIRCLE ( 'NONE', #5241, 5.000000000000004441 ) ;
#2809=CARTESIAN_POINT ( 'NONE',  ( 114.9999999999999147, 99.99999999999998579, 250.0000000000000000 ) ) ;
#2813=LINE ( 'NONE', #720, #7936 ) ;
#2828=EDGE_CURVE ( 'NONE', #4917, #2993, #913, .T. ) ;
#2832=EDGE_LOOP ( 'NONE', ( #4045, #7731 ) ) ;
#2835=EDGE_CURVE ( 'NONE', #6124, #8026, #3416, .T. ) ;
#2838=DIRECTION ( 'NONE',  ( -1.000000000000000000, 0.000000000000000000, 0.000000000000000000 ) ) ;
#2844=ORIENTED_EDGE ( 'NONE', *, *, #1046, .F. ) ;
#2865=EDGE_CURVE ( 'NONE', #2040, #7952, #4139, .T. ) ;
#2867=AXIS2_PLACEMENT_3D ( 'NONE', #7664, #5113, #1246 ) ;
#2873=ORIENTED_EDGE ( 'NONE', *, *, #5607, .T. ) ;
#2874=CARTESIAN_POINT ( 'NONE',  ( -120.9999999999999005, -115.0000000000000000, 8.205133554287239938E-16 ) ) ;
#2881=ORIENTED_EDGE ( 'NONE', *, *, #4940, .T. ) ;
#2888=EDGE_LOOP ( 'NONE', ( #6207, #3803, #4865, #5544 ) ) ;
#2900=CARTESIAN_POINT ( 'NONE',  ( 15.00000000000000355, 0.000000000000000000, -118.0000000000000284 ) ) ;
#2902=ORIENTED_EDGE ( 'NONE', *, *, #180, .T. ) ;
#2903=CARTESIAN_POINT ( 'NONE',  ( 120.9999999999999005, 115.0000000000000000, 8.205133554287239938E-16 ) ) ;
#2917=VECTOR ( 'NONE', #1174, 1000.000000000000000 ) ;
#2918=VERTEX_POINT ( 'NONE', #959 ) ;
#2920=FACE_BOUND ( 'NONE', #5205, .T. ) ;
#2929=( LENGTH_UNIT ( ) NAMED_UNIT ( * ) SI_UNIT ( .MILLI., .METRE. ) );
#2930=CIRCLE ( 'NONE', #3460, 15.00000000000000178 ) ;
#2935=CARTESIAN_POINT ( 'NONE',  ( 25.00000000000000000, 3.061616997868383043E-15, -126.0000000000000284 ) ) ;
#2940=ADVANCED_FACE ( 'NONE', ( #2137 ), #2743, .T. ) ;
#2947=DIRECTION ( 'NONE',  ( -0.000000000000000000, -0.000000000000000000, -1.000000000000000000 ) ) ;
#2955=AXIS2_PLACEMENT_3D ( 'NONE', #6274, #7509, #7986 ) ;
#2962=CARTESIAN_POINT ( 'NONE',  ( -15.00000000000000000, 1.836970198721029589E-15, -128.0000000000000284 ) ) ;
#2964=EDGE_CURVE ( 'NONE', #6525, #4104, #3083, .T. ) ;
#2969=DIRECTION ( 'NONE',  ( -0.000000000000000000, -0.000000000000000000, 1.000000000000000000 ) ) ;
#2980=ORIENTED_EDGE ( 'NONE', *, *, #6601, .T. ) ;
#2993=VERTEX_POINT ( 'NONE', #5021 ) ;
#2995=DIRECTION ( 'NONE',  ( 1.000000000000000000, 0.000000000000000000, 0.000000000000000000 ) ) ;
#2996=ORIENTED_EDGE ( 'NONE', *, *, #308, .T. ) ;
#2998=CARTESIAN_POINT ( 'NONE',  ( -120.0000000000000000, -120.0000000000000000, -28.00000000000002487 ) ) ;
#3000=VERTEX_POINT ( 'NONE', #6287 ) ;
#3002=VECTOR ( 'NONE', #7020, 1000.000000000000000 ) ;
#3006=DIRECTION ( 'NONE',  ( 0.000000000000000000, 1.000000000000000000, 0.000000000000000000 ) ) ;
#3014=STYLED_ITEM('',(#8393),#706);
#3015=VERTEX_POINT ( 'NONE', #2467 ) ;
#3016=EDGE_LOOP ( 'NONE', ( #3304, #7912 ) ) ;
#3026=CARTESIAN_POINT ( 'NONE',  ( 0.000000000000000000, 0.000000000000000000, -128.0000000000000284 ) ) ;
#3027=DIRECTION ( 'NONE',  ( -1.000000000000000000, 0.000000000000000000, 0.000000000000000000 ) ) ;
#3031=EDGE_LOOP ( 'NONE', ( #2568, #5226, #7519, #4754 ) ) ;
#3039=ORIENTED_EDGE ( 'NONE', *, *, #2471, .T. ) ;
#3040=AXIS2_PLACEMENT_3D ( 'NONE', #5707, #2591, #7660 ) ;
#3063=DIRECTION ( 'NONE',  ( 0.000000000000000000, -0.000000000000000000, -1.000000000000000000 ) ) ;
#3068=AXIS2_PLACEMENT_3D ( 'NONE', #2422, #7395, #5617 ) ;
#3082=CYLINDRICAL_SURFACE ( 'NONE', #2169, 5.999999999999991118 ) ;
#3083=LINE ( 'NONE', #3231, #8055 ) ;
#3097=CIRCLE ( 'NONE', #3485, 15.00000000000001421 ) ;
#3102=CARTESIAN_POINT ( 'NONE',  ( 17.61817604250836311, 0.000000000000000000, -120.5000000000000284 ) ) ;
#3133=EDGE_CURVE ( 'NONE', #1787, #1402, #1056, .T. ) ;
#3138=CARTESIAN_POINT ( 'NONE',  ( 125.0000000000000000, -125.0000000000000000, 0.000000000000000000 ) ) ;
#3146=VERTEX_POINT ( 'NONE', #3465 ) ;
#3149=EDGE_LOOP ( 'NONE', ( #2844, #4219 ) ) ;
#3150=CARTESIAN_POINT ( 'NONE',  ( 99.99999999999991473, -115.0000000000000000, 250.0000000000000000 ) ) ;
#3159=DIRECTION ( 'NONE',  ( 0.000000000000000000, 0.000000000000000000, 1.000000000000000000 ) ) ;
#3161=CARTESIAN_POINT ( 'NONE',  ( 14.30908802125418511, 4.500000000000000000, -126.0000000000000284 ) ) ;
#3162=CARTESIAN_POINT ( 'NONE',  ( 114.9999999999999147, -115.0000000000000000, 250.0000000000000000 ) ) ;
#3190=EDGE_LOOP ( 'NONE', ( #7937, #1108 ) ) ;
#3192=CARTESIAN_POINT ( 'NONE',  ( -120.0000000000000000, -125.0000000000000000, -28.00000000000002487 ) ) ;
#3196=ORIENTED_EDGE ( 'NONE', *, *, #6952, .T. ) ;
#3201=ORIENTED_EDGE ( 'NONE', *, *, #6275, .F. ) ;
#3208=VECTOR ( 'NONE', #5178, 1000.000000000000000 ) ;
#3212=APPLICATION_CONTEXT ( 'automotive_design' ) ;
#3219=AXIS2_PLACEMENT_3D ( 'NONE', #300, #7958, #7320 ) ;
#3224=ORIENTED_EDGE ( 'NONE', *, *, #1745, .T. ) ;
#3228=CYLINDRICAL_SURFACE ( 'NONE', #5653, 5.999999999999991118 ) ;
#3231=CARTESIAN_POINT ( 'NONE',  ( 108.9999999999999147, 115.0000000000000000, 0.000000000000000000 ) ) ;
#3239=CARTESIAN_POINT ( 'NONE',  ( 17.61817604250836311, -4.500000000000000000, -126.0000000000000284 ) ) ;
#3251=LINE ( 'NONE', #5916, #7651 ) ;
#3254=ORIENTED_EDGE ( 'NONE', *, *, #991, .F. ) ;
#3260=PRODUCT_DEFINITION_FORMATION_WITH_SPECIFIED_SOURCE ( 'ANY', '', #7894, .NOT_KNOWN. ) ;
#3265=ORIENTED_EDGE ( 'NONE', *, *, #3764, .T. ) ;
#3267=VERTEX_POINT ( 'NONE', #6132 ) ;
#3276=ORIENTED_EDGE ( 'NONE', *, *, #1646, .F. ) ;
#3287=DIRECTION ( 'NONE',  ( -1.000000000000000000, 0.000000000000000000, 0.000000000000000000 ) ) ;
#3296=ADVANCED_FACE ( 'NONE', ( #2283 ), #4223, .F. ) ;
#3299=EDGE_LOOP ( 'NONE', ( #7878, #8141 ) ) ;
#3300=ORIENTED_EDGE ( 'NONE', *, *, #4940, .F. ) ;
#3304=ORIENTED_EDGE ( 'NONE', *, *, #5622, .F. ) ;
#3308=DIRECTION ( 'NONE',  ( 1.000000000000000000, 0.000000000000000000, 0.000000000000000000 ) ) ;
#3320=AXIS2_PLACEMENT_3D ( 'NONE', #1886, #2633, #6460 ) ;
#3328=LINE ( 'NONE', #7277, #4383 ) ;
#3335=VECTOR ( 'NONE', #5390, 1000.000000000000000 ) ;
#3336=AXIS2_PLACEMENT_3D ( 'NONE', #6918, #493, #6481 ) ;
#3337=DIRECTION ( 'NONE',  ( 0.000000000000000000, -0.000000000000000000, -1.000000000000000000 ) ) ;
#3341=CIRCLE ( 'NONE', #7947, 5.999999999999991118 ) ;
#3342=AXIS2_PLACEMENT_3D ( 'NONE', #1151, #1739, #8110 ) ;
#3346=CYLINDRICAL_SURFACE ( 'NONE', #583, 5.999999999999991118 ) ;
#3358=CARTESIAN_POINT ( 'NONE',  ( 14.30908802125418511, 4.500000000000000000, -118.0000000000000284 ) ) ;
#3365=FACE_OUTER_BOUND ( 'NONE', #705, .T. ) ;
#3369=DIRECTION ( 'NONE',  ( 0.000000000000000000, 0.000000000000000000, -1.000000000000000000 ) ) ;
#3370=CIRCLE ( 'NONE', #6486, 5.999999999999991118 ) ;
#3377=DIRECTION ( 'NONE',  ( -0.000000000000000000, -0.000000000000000000, -1.000000000000000000 ) ) ;
#3382=DIRECTION ( 'NONE',  ( -0.000000000000000000, -0.000000000000000000, 1.000000000000000000 ) ) ;
#3396=CARTESIAN_POINT ( 'NONE',  ( -125.0000000000000000, 120.0000000000000000, 0.000000000000000000 ) ) ;
#3399=CARTESIAN_POINT ( 'NONE',  ( 99.99999999999991473, -115.0000000000000000, 0.000000000000000000 ) ) ;
#3413=DIRECTION ( 'NONE',  ( 1.000000000000000000, 0.000000000000000000, 0.000000000000000000 ) ) ;
#3416=LINE ( 'NONE', #217, #2273 ) ;
#3417=ORIENTED_EDGE ( 'NONE', *, *, #190, .T. ) ;
#3418=CARTESIAN_POINT ( 'NONE',  ( 120.0000000000000000, -120.0000000000000000, 0.000000000000000000 ) ) ;
#3419=EDGE_CURVE ( 'NONE', #5233, #698, #3454, .T. ) ;
#3420=ADVANCED_FACE ( 'NONE', ( #6044 ), #5998, .F. ) ;
#3434=VECTOR ( 'NONE', #3413, 1000.000000000000000 ) ;
#3439=EDGE_CURVE ( 'NONE', #1787, #4917, #744, .T. ) ;
#3445=DIRECTION ( 'NONE',  ( -0.000000000000000000, -0.000000000000000000, 1.000000000000000000 ) ) ;
#3447=ORIENTED_EDGE ( 'NONE', *, *, #6227, .T. ) ;
#3454=LINE ( 'NONE', #3941, #3434 ) ;
#3460=AXIS2_PLACEMENT_3D ( 'NONE', #1521, #4075, #6663 ) ;
#3465=CARTESIAN_POINT ( 'NONE',  ( 120.0000000000000000, -125.0000000000000000, 0.000000000000000000 ) ) ;
#3468=ADVANCED_FACE ( 'NONE', ( #2753, #7846 ), #4613, .F. ) ;
#3475=ORIENTED_EDGE ( 'NONE', *, *, #4100, .T. ) ;
#3479=DIRECTION ( 'NONE',  ( -0.000000000000000000, -0.000000000000000000, -1.000000000000000000 ) ) ;
#3483=DIRECTION ( 'NONE',  ( -0.000000000000000000, -0.000000000000000000, 1.000000000000000000 ) ) ;
#3485=AXIS2_PLACEMENT_3D ( 'NONE', #430, #5712, #8334 ) ;
#3493=ORIENTED_EDGE ( 'NONE', *, *, #3639, .T. ) ;
#3502=ORIENTED_EDGE ( 'NONE', *, *, #2640, .T. ) ;
#3517=DIRECTION ( 'NONE',  ( 0.000000000000000000, -0.000000000000000000, -1.000000000000000000 ) ) ;
#3526=DIRECTION ( 'NONE',  ( -0.000000000000000000, -0.000000000000000000, 1.000000000000000000 ) ) ;
#3527=CARTESIAN_POINT ( 'NONE',  ( 17.61817604250836311, 4.500000000000000000, -118.0000000000000284 ) ) ;
#3535=FACE_OUTER_BOUND ( 'NONE', #4398, .T. ) ;
#3540=( LENGTH_UNIT ( ) NAMED_UNIT ( * ) SI_UNIT ( .MILLI., .METRE. ) );
#3550=PLANE ( 'NONE',  #7826 ) ;
#3557=ORIENTED_EDGE ( 'NONE', *, *, #5585, .F. ) ;
#3580=CARTESIAN_POINT ( 'NONE',  ( 120.9999999999999005, -115.0000000000000000, 8.205133554287239938E-16 ) ) ;
#3591=FACE_BOUND ( 'NONE', #4303, .T. ) ;
#3593=DIRECTION ( 'NONE',  ( 0.000000000000000000, -1.000000000000000000, 0.000000000000000000 ) ) ;
#3596=DIRECTION ( 'NONE',  ( -0.000000000000000000, -0.000000000000000000, 1.000000000000000000 ) ) ;
#3602=VERTEX_POINT ( 'NONE', #5632 ) ;
#3605=AXIS2_PLACEMENT_3D ( 'NONE', #1513, #5270, #6654 ) ;
#3609=ORIENTED_EDGE ( 'NONE', *, *, #7662, .T. ) ;
#3612=VECTOR ( 'NONE', #1170, 1000.000000000000000 ) ;
#3613=AXIS2_PLACEMENT_3D ( 'NONE', #5955, #4646, #4686 ) ;
#3614=EDGE_LOOP ( 'NONE', ( #2491, #1891, #3224, #1220 ) ) ;
#3619=DIRECTION ( 'NONE',  ( 0.000000000000000000, -1.000000000000000000, 0.000000000000000000 ) ) ;
#3623=CARTESIAN_POINT ( 'NONE',  ( -114.9999999999999147, -115.0000000000000000, -28.00000000000002487 ) ) ;
#3627=CARTESIAN_POINT ( 'NONE',  ( 0.000000000000000000, 4.500000000000000000, -120.5000000000000284 ) ) ;
#3628=EDGE_CURVE ( 'NONE', #3712, #5309, #8214, .T. ) ;
#3634=ORIENTED_EDGE ( 'NONE', *, *, #3439, .F. ) ;
#3635=EDGE_CURVE ( 'NONE', #2291, #441, #5330, .T. ) ;
#3636=DIRECTION ( 'NONE',  ( 1.000000000000000000, 0.000000000000000000, 0.000000000000000000 ) ) ;
#3639=EDGE_CURVE ( 'NONE', #8098, #3712, #7790, .T. ) ;
#3642=ORIENTED_EDGE ( 'NONE', *, *, #7323, .T. ) ;
#3645=ORIENTED_EDGE ( 'NONE', *, *, #7990, .T. ) ;
#3649=ADVANCED_FACE ( 'NONE', ( #2675 ), #2140, .T. ) ;
#3653=EDGE_CURVE ( 'NONE', #381, #5233, #3251, .T. ) ;
#3664=CARTESIAN_POINT ( 'NONE',  ( 0.000000000000000000, 115.0000000000000000, 0.000000000000000000 ) ) ;
#3666=ADVANCED_FACE ( 'NONE', ( #7876 ), #776, .T. ) ;
#3667=FACE_OUTER_BOUND ( 'NONE', #433, .T. ) ;
#3669=DIRECTION ( 'NONE',  ( -0.000000000000000000, -0.000000000000000000, -1.000000000000000000 ) ) ;
#3671=EDGE_LOOP ( 'NONE', ( #8197, #1178, #6435, #2531 ) ) ;
#3683=DIRECTION ( 'NONE',  ( -0.000000000000000000, -0.000000000000000000, 1.000000000000000000 ) ) ;
#3684=CIRCLE ( 'NONE', #8142, 5.999999999999991118 ) ;
#3687=PLANE ( 'NONE',  #5247 ) ;
#3692=CARTESIAN_POINT ( 'NONE',  ( 0.000000000000000000, 0.000000000000000000, -128.0000000000000284 ) ) ;
#3693=EDGE_CURVE ( 'NONE', #6430, #2575, #3328, .T. ) ;
#3699=CARTESIAN_POINT ( 'NONE',  ( 114.9999999999999147, 115.0000000000000000, 0.000000000000000000 ) ) ;
#3703=CARTESIAN_POINT ( 'NONE',  ( -125.0000000000000000, -125.0000000000000000, 0.000000000000000000 ) ) ;
#3712=VERTEX_POINT ( 'NONE', #7840 ) ;
#3713=DIRECTION ( 'NONE',  ( -0.000000000000000000, -0.000000000000000000, 1.000000000000000000 ) ) ;
#3721=DIRECTION ( 'NONE',  ( -1.000000000000000000, 0.000000000000000000, 0.000000000000000000 ) ) ;
#3733=FACE_OUTER_BOUND ( 'NONE', #2403, .T. ) ;
#3735=DIRECTION ( 'NONE',  ( 1.000000000000000000, 0.000000000000000000, 0.000000000000000000 ) ) ;
#3738=CARTESIAN_POINT ( 'NONE',  ( 0.000000000000000000, -4.500000000000000000, -120.5000000000000284 ) ) ;
#3739=VERTEX_POINT ( 'NONE', #2903 ) ;
#3740=VECTOR ( 'NONE', #3889, 1000.000000000000000 ) ;
#3744=FACE_OUTER_BOUND ( 'NONE', #4171, .T. ) ;
#3751=ORIENTED_EDGE ( 'NONE', *, *, #6547, .T. ) ;
#3757=AXIS2_PLACEMENT_3D ( 'NONE', #506, #2464, #3159 ) ;
#3764=EDGE_CURVE ( 'NONE', #1618, #4405, #4117, .T. ) ;
#3772=AXIS2_PLACEMENT_3D ( 'NONE', #6117, #2308, #2233 ) ;
#3785=CARTESIAN_POINT ( 'NONE',  ( 17.61817604250836311, 0.000000000000000000, -128.0000000000000284 ) ) ;
#3788=ORIENTED_EDGE ( 'NONE', *, *, #8093, .T. ) ;
#3803=ORIENTED_EDGE ( 'NONE', *, *, #2585, .F. ) ;
#3805=VECTOR ( 'NONE', #3027, 1000.000000000000000 ) ;
#3827=EDGE_CURVE ( 'NONE', #441, #7933, #1139, .T. ) ;
#3830=CARTESIAN_POINT ( 'NONE',  ( -108.9999999999999147, -115.0000000000000000, 8.205133554287239938E-16 ) ) ;
#3836=ORIENTED_EDGE ( 'NONE', *, *, #7528, .T. ) ;
#3840=DIRECTION ( 'NONE',  ( 1.000000000000000000, 0.000000000000000000, 0.000000000000000000 ) ) ;
#3844=DIRECTION ( 'NONE',  ( 1.000000000000000000, 0.000000000000000000, 0.000000000000000000 ) ) ;
#3863=DIRECTION ( 'NONE',  ( -0.000000000000000000, -0.000000000000000000, 1.000000000000000000 ) ) ;
#3865=VECTOR ( 'NONE', #3006, 1000.000000000000000 ) ;
#3867=VERTEX_POINT ( 'NONE', #1925 ) ;
#3881=ORIENTED_EDGE ( 'NONE', *, *, #5404, .T. ) ;
#3887=AXIS2_PLACEMENT_3D ( 'NONE', #7785, #6584, #3962 ) ;
#3889=DIRECTION ( 'NONE',  ( 0.000000000000000000, 1.000000000000000000, -0.000000000000000000 ) ) ;
#3891=CIRCLE ( 'NONE', #1338, 14.99999999999998579 ) ;
#3894=ORIENTED_EDGE ( 'NONE', *, *, #7029, .T. ) ;
#3898=ORIENTED_EDGE ( 'NONE', *, *, #4753, .F. ) ;
#3908=ORIENTED_EDGE ( 'NONE', *, *, #3639, .F. ) ;
#3909=EDGE_CURVE ( 'NONE', #4158, #6525, #6293, .T. ) ;
#3911=VECTOR ( 'NONE', #6678, 1000.000000000000000 ) ;
#3940=DIRECTION ( 'NONE',  ( -1.000000000000000000, 0.000000000000000000, 0.000000000000000000 ) ) ;
#3941=CARTESIAN_POINT ( 'NONE',  ( -125.0000000000000000, 125.0000000000000000, 0.000000000000000000 ) ) ;
#3950=EDGE_CURVE ( 'NONE', #7585, #805, #5925, .T. ) ;
#3961=EDGE_CURVE ( 'NONE', #3000, #306, #1315, .T. ) ;
#3962=DIRECTION ( 'NONE',  ( -1.000000000000000000, 0.000000000000000000, 0.000000000000000000 ) ) ;
#3975=VECTOR ( 'NONE', #6251, 1000.000000000000000 ) ;
#4000=ADVANCED_FACE ( 'NONE', ( #1036, #2920, #3591, #2396, #5680, #1764 ), #1712, .T. ) ;
#4001=ADVANCED_FACE ( 'NONE', ( #4906 ), #1843, .F. ) ;
#4004=FACE_OUTER_BOUND ( 'NONE', #6458, .T. ) ;
#4007=ORIENTED_EDGE ( 'NONE', *, *, #3950, .F. ) ;
#4028=DIRECTION ( 'NONE',  ( 0.000000000000000000, 1.000000000000000000, -0.000000000000000000 ) ) ;
#4035=CARTESIAN_POINT ( 'NONE',  ( -120.0000000000000000, 125.0000000000000000, 0.000000000000000000 ) ) ;
#4041=DIRECTION ( 'NONE',  ( 0.000000000000000000, -1.000000000000000000, 0.000000000000000000 ) ) ;
#4045=ORIENTED_EDGE ( 'NONE', *, *, #2298, .F. ) ;
#4054=PLANE ( 'NONE',  #2355 ) ;
#4057=DIRECTION ( 'NONE',  ( 1.000000000000000000, 0.000000000000000000, 0.000000000000000000 ) ) ;
#4058=EDGE_CURVE ( 'NONE', #1522, #3867, #5553, .T. ) ;
#4070=DIRECTION ( 'NONE',  ( -0.000000000000000000, -0.000000000000000000, 1.000000000000000000 ) ) ;
#4073=ADVANCED_FACE ( 'NONE', ( #8173 ), #5513, .F. ) ;
#4074=EDGE_LOOP ( 'NONE', ( #4626, #7759, #7468, #4207, #6058 ) ) ;
#4075=DIRECTION ( 'NONE',  ( 0.000000000000000000, 0.000000000000000000, -1.000000000000000000 ) ) ;
#4095=DIRECTION ( 'NONE',  ( 0.000000000000000000, -0.000000000000000000, -1.000000000000000000 ) ) ;
#4100=EDGE_CURVE ( 'NONE', #4405, #6401, #1039, .T. ) ;
#4103=CARTESIAN_POINT ( 'NONE',  ( -114.9999999999999147, 0.000000000000000000, 250.0000000000000000 ) ) ;
#4104=VERTEX_POINT ( 'NONE', #1332 ) ;
#4109=LINE ( 'NONE', #6096, #2197 ) ;
#4111=VECTOR ( 'NONE', #261, 1000.000000000000000 ) ;
#4115=ORIENTED_EDGE ( 'NONE', *, *, #7990, .F. ) ;
#4117=LINE ( 'NONE', #934, #4670 ) ;
#4118=AXIS2_PLACEMENT_3D ( 'NONE', #5841, #7795, #2711 ) ;
#4126=CYLINDRICAL_SURFACE ( 'NONE', #3613, 15.00000000000001421 ) ;
#4128=ORIENTED_EDGE ( 'NONE', *, *, #3653, .T. ) ;
#4133=DIRECTION ( 'NONE',  ( -0.000000000000000000, -0.000000000000000000, -1.000000000000000000 ) ) ;
#4137=SHAPE_REPRESENTATION_RELATIONSHIP ( 'NONE' , 'NONE' ,  #1440, #6626 ) ;
#4139=LINE ( 'NONE', #2797, #1322 ) ;
#4149=( NAMED_UNIT ( * ) SI_UNIT ( $, .STERADIAN. ) SOLID_ANGLE_UNIT ( ) );
#4153=ORIENTED_EDGE ( 'NONE', *, *, #5585, .T. ) ;
#4158=VERTEX_POINT ( 'NONE', #8 ) ;
#4171=EDGE_LOOP ( 'NONE', ( #748, #1714, #5862, #2303 ) ) ;
#4174=CARTESIAN_POINT ( 'NONE',  ( -114.9999999999999147, 115.0000000000000000, -28.00000000000002487 ) ) ;
#4175=ORIENTED_EDGE ( 'NONE', *, *, #6765, .F. ) ;
#4178=FACE_OUTER_BOUND ( 'NONE', #5643, .T. ) ;
#4182=VERTEX_POINT ( 'NONE', #7843 ) ;
#4184=DIRECTION ( 'NONE',  ( 1.000000000000000000, 0.000000000000000000, 0.000000000000000000 ) ) ;
#4186=DIRECTION ( 'NONE',  ( -1.000000000000000000, 0.000000000000000000, 0.000000000000000000 ) ) ;
#4190=DIRECTION ( 'NONE',  ( 1.000000000000000000, 0.000000000000000000, 0.000000000000000000 ) ) ;
#4196=DIRECTION ( 'NONE',  ( -0.000000000000000000, 0.000000000000000000, 1.000000000000000000 ) ) ;
#4204=EDGE_CURVE ( 'NONE', #5510, #5315, #741, .T. ) ;
#4206=VERTEX_POINT ( 'NONE', #2561 ) ;
#4207=ORIENTED_EDGE ( 'NONE', *, *, #735, .T. ) ;
#4210=DIRECTION ( 'NONE',  ( 1.000000000000000000, 0.000000000000000000, 0.000000000000000000 ) ) ;
#4215=ORIENTED_EDGE ( 'NONE', *, *, #198, .F. ) ;
#4219=ORIENTED_EDGE ( 'NONE', *, *, #5928, .F. ) ;
#4220=DIRECTION ( 'NONE',  ( 1.000000000000000000, 0.000000000000000000, 0.000000000000000000 ) ) ;
#4222=FACE_OUTER_BOUND ( 'NONE', #4694, .T. ) ;
#4223=CYLINDRICAL_SURFACE ( 'NONE', #8037, 5.999999999999991118 ) ;
#4229=ORIENTED_EDGE ( 'NONE', *, *, #4058, .F. ) ;
#4238=VECTOR ( 'NONE', #7804, 1000.000000000000000 ) ;
#4239=ORIENTED_EDGE ( 'NONE', *, *, #2141, .F. ) ;
#4249=LINE ( 'NONE', #5628, #2620 ) ;
#4254=EDGE_CURVE ( 'NONE', #2918, #7952, #1215, .T. ) ;
#4257=VECTOR ( 'NONE', #2511, 1000.000000000000000 ) ;
#4268=ORIENTED_EDGE ( 'NONE', *, *, #4523, .F. ) ;
#4284=PLANE ( 'NONE',  #3068 ) ;
#4286=CARTESIAN_POINT ( 'NONE',  ( 114.9999999999999147, 115.0000000000000000, 0.000000000000000000 ) ) ;
#4289=VECTOR ( 'NONE', #2055, 1000.000000000000000 ) ;
#4300=ORIENTED_EDGE ( 'NONE', *, *, #7602, .T. ) ;
#4303=EDGE_LOOP ( 'NONE', ( #4883, #3609 ) ) ;
#4304=DIRECTION ( 'NONE',  ( 1.000000000000000000, 0.000000000000000000, 0.000000000000000000 ) ) ;
#4306=CYLINDRICAL_SURFACE ( 'NONE', #4493, 5.000000000000004441 ) ;
#4313=CARTESIAN_POINT ( 'NONE',  ( -114.9999999999999147, -100.0000000000000000, 250.0000000000000000 ) ) ;
#4333=ORIENTED_EDGE ( 'NONE', *, *, #2865, .T. ) ;
#4355=AXIS2_PLACEMENT_3D ( 'NONE', #4570, #3619, #3337 ) ;
#4379=VERTEX_POINT ( 'NONE', #5332 ) ;
#4381=EDGE_CURVE ( 'NONE', #7564, #900, #8331, .T. ) ;
#4383=VECTOR ( 'NONE', #2746, 1000.000000000000000 ) ;
#4386=VERTEX_POINT ( 'NONE', #7233 ) ;
#4394=DIRECTION ( 'NONE',  ( 1.000000000000000000, 0.000000000000000000, 0.000000000000000000 ) ) ;
#4398=EDGE_LOOP ( 'NONE', ( #1055, #1223 ) ) ;
#4402=DIRECTION ( 'NONE',  ( 1.000000000000000000, 0.000000000000000000, 0.000000000000000000 ) ) ;
#4405=VERTEX_POINT ( 'NONE', #827 ) ;
#4408=CIRCLE ( 'NONE', #5097, 5.999999999999991118 ) ;
#4409=ORIENTED_EDGE ( 'NONE', *, *, #7798, .T. ) ;
#4417=EDGE_CURVE ( 'NONE', #6215, #3867, #1794, .T. ) ;
#4459=FACE_OUTER_BOUND ( 'NONE', #3671, .T. ) ;
#4469=ADVANCED_FACE ( 'NONE', ( #475 ), #4941, .T. ) ;
#4470=CARTESIAN_POINT ( 'NONE',  ( 120.9999999999999005, -115.0000000000000000, -28.00000000000002487 ) ) ;
#4472=VECTOR ( 'NONE', #6027, 1000.000000000000000 ) ;
#4474=ORIENTED_EDGE ( 'NONE', *, *, #4685, .T. ) ;
#4489=ORIENTED_EDGE ( 'NONE', *, *, #5623, .T. ) ;
#4493=AXIS2_PLACEMENT_3D ( 'NONE', #6906, #7588, #4220 ) ;
#4507=CARTESIAN_POINT ( 'NONE',  ( 0.000000000000000000, 0.000000000000000000, -120.5000000000000284 ) ) ;
#4514=ORIENTED_EDGE ( 'NONE', *, *, #5475, .F. ) ;
#4516=AXIS2_PLACEMENT_3D ( 'NONE', #786, #7847, #4057 ) ;
#4523=EDGE_CURVE ( 'NONE', #3267, #326, #4900, .T. ) ;
#4529=ORIENTED_EDGE ( 'NONE', *, *, #2865, .F. ) ;
#4531=EDGE_LOOP ( 'NONE', ( #6257, #6007, #1776, #1992 ) ) ;
#4542=ORIENTED_EDGE ( 'NONE', *, *, #4417, .F. ) ;
#4560=DIRECTION ( 'NONE',  ( -0.000000000000000000, -0.000000000000000000, -1.000000000000000000 ) ) ;
#4570=CARTESIAN_POINT ( 'NONE',  ( 0.000000000000000000, 4.500000000000000000, -128.0000000000000284 ) ) ;
#4594=ORIENTED_EDGE ( 'NONE', *, *, #735, .F. ) ;
#4601=CARTESIAN_POINT ( 'NONE',  ( 17.61817604250836311, -4.500000000000000000, -128.0000120000000265 ) ) ;
#4606=DIRECTION ( 'NONE',  ( -0.000000000000000000, 0.000000000000000000, 1.000000000000000000 ) ) ;
#4610=DIRECTION ( 'NONE',  ( 1.000000000000000000, 0.000000000000000000, 0.000000000000000000 ) ) ;
#4611=CARTESIAN_POINT ( 'NONE',  ( 120.0000000000000000, 125.0000000000000000, 0.000000000000000000 ) ) ;
#4613=PLANE ( 'NONE',  #753 ) ;
#4626=ORIENTED_EDGE ( 'NONE', *, *, #5261, .F. ) ;
#4628=DIRECTION ( 'NONE',  ( 1.000000000000000000, 0.000000000000000000, 0.000000000000000000 ) ) ;
#4633=EDGE_CURVE ( 'NONE', #1402, #6246, #644, .T. ) ;
#4644=DIRECTION ( 'NONE',  ( -1.000000000000000000, 0.000000000000000000, 0.000000000000000000 ) ) ;
#4646=DIRECTION ( 'NONE',  ( -0.000000000000000000, -0.000000000000000000, -1.000000000000000000 ) ) ;
#4649=DIRECTION ( 'NONE',  ( -1.000000000000000000, 0.000000000000000000, -0.000000000000000000 ) ) ;
#4651=EDGE_CURVE ( 'NONE', #3712, #5164, #5833, .T. ) ;
#4653=CARTESIAN_POINT ( 'NONE',  ( 114.9999999999999147, -115.0000000000000000, 8.205133554287239938E-16 ) ) ;
#4670=VECTOR ( 'NONE', #3483, 1000.000000000000000 ) ;
#4676=EDGE_CURVE ( 'NONE', #1010, #5315, #1457, .T. ) ;
#4679=AXIS2_PLACEMENT_3D ( 'NONE', #2706, #2102, #4644 ) ;
#4681=CARTESIAN_POINT ( 'NONE',  ( -108.9999999999999147, 115.0000000000000000, 0.000000000000000000 ) ) ;
#4685=EDGE_CURVE ( 'NONE', #4182, #6124, #8293, .T. ) ;
#4686=DIRECTION ( 'NONE',  ( -1.000000000000000000, 0.000000000000000000, 0.000000000000000000 ) ) ;
#4694=EDGE_LOOP ( 'NONE', ( #5690, #4239, #2455, #3642, #1602, #6527, #4948, #6942, #2629, #7654 ) ) ;
#4697=CIRCLE ( 'NONE', #7678, 15.00000000000000000 ) ;
#4712=CARTESIAN_POINT ( 'NONE',  ( -99.99999999999990052, 115.0000000000000000, 0.000000000000000000 ) ) ;
#4714=VECTOR ( 'NONE', #4402, 1000.000000000000000 ) ;
#4716=CARTESIAN_POINT ( 'NONE',  ( -120.0000000000000000, 120.0000000000000000, -28.00000000000002487 ) ) ;
#4726=CARTESIAN_POINT ( 'NONE',  ( 125.0000000000000000, -120.0000000000000000, -28.00000000000002487 ) ) ;
#4728=ORIENTED_EDGE ( 'NONE', *, *, #875, .T. ) ;
#4746=CARTESIAN_POINT ( 'NONE',  ( -114.9999999999999147, -115.0000000000000000, 0.000000000000000000 ) ) ;
#4753=EDGE_CURVE ( 'NONE', #2097, #179, #5953, .T. ) ;
#4754=ORIENTED_EDGE ( 'NONE', *, *, #6791, .T. ) ;
#4763=CARTESIAN_POINT ( 'NONE',  ( 14.30908802125418511, -4.500000000000000000, -128.0000000000000284 ) ) ;
#4768=( GEOMETRIC_REPRESENTATION_CONTEXT ( 3 ) GLOBAL_UNCERTAINTY_ASSIGNED_CONTEXT ( ( #6745 ) ) GLOBAL_UNIT_ASSIGNED_CONTEXT ( ( #2929, #1558, #4149 ) ) REPRESENTATION_CONTEXT ( 'NONE', 'WORKASPACE' ) );
#4769=ORIENTED_EDGE ( 'NONE', *, *, #4254, .F. ) ;
#4782=ORIENTED_EDGE ( 'NONE', *, *, #4881, .F. ) ;
#4809=ORIENTED_EDGE ( 'NONE', *, *, #6866, .T. ) ;
#4812=EDGE_LOOP ( 'NONE', ( #29, #8137, #6970, #3898 ) ) ;
#4837=EDGE_CURVE ( 'NONE', #5309, #4868, #8338, .T. ) ;
#4842=ORIENTED_EDGE ( 'NONE', *, *, #2768, .F. ) ;
#4847=CARTESIAN_POINT ( 'NONE',  ( 0.000000000000000000, 0.000000000000000000, 250.0000000000000000 ) ) ;
#4849=CARTESIAN_POINT ( 'NONE',  ( 14.30908802125418511, -4.500000000000000000, -120.5000000000000284 ) ) ;
#4854=DIRECTION ( 'NONE',  ( -0.000000000000000000, -0.000000000000000000, 1.000000000000000000 ) ) ;
#4857=DIRECTION ( 'NONE',  ( 0.000000000000000000, 0.000000000000000000, -1.000000000000000000 ) ) ;
#4860=ORIENTED_EDGE ( 'NONE', *, *, #1135, .F. ) ;
#4865=ORIENTED_EDGE ( 'NONE', *, *, #570, .T. ) ;
#4868=VERTEX_POINT ( 'NONE', #465 ) ;
#4872=EDGE_CURVE ( 'NONE', #5616, #5541, #2377, .T. ) ;
#4881=EDGE_CURVE ( 'NONE', #3015, #6124, #5577, .T. ) ;
#4883=ORIENTED_EDGE ( 'NONE', *, *, #3909, .T. ) ;
#4889=ORIENTED_EDGE ( 'NONE', *, *, #5623, .F. ) ;
#4891=CIRCLE ( 'NONE', #1259, 15.00000000000001421 ) ;
#4895=FACE_OUTER_BOUND ( 'NONE', #7516, .T. ) ;
#4897=ORIENTED_EDGE ( 'NONE', *, *, #2685, .T. ) ;
#4900=LINE ( 'NONE', #7491, #911 ) ;
#4901=LINE ( 'NONE', #6726, #2050 ) ;
#4906=FACE_OUTER_BOUND ( 'NONE', #859, .T. ) ;
#4909=ORIENTED_EDGE ( 'NONE', *, *, #1439, .F. ) ;
#4912=CIRCLE ( 'NONE', #6129, 5.000000000000004441 ) ;
#4913=ORIENTED_EDGE ( 'NONE', *, *, #7184, .T. ) ;
#4917=VERTEX_POINT ( 'NONE', #6793 ) ;
#4929=ADVANCED_FACE ( 'NONE', ( #3667 ), #4284, .T. ) ;
#4939=AXIS2_PLACEMENT_3D ( 'NONE', #6933, #8245, #7613 ) ;
#4940=EDGE_CURVE ( 'NONE', #6868, #6215, #6025, .T. ) ;
#4941=CYLINDRICAL_SURFACE ( 'NONE', #2789, 5.000000000000004441 ) ;
#4942=PLANE ( 'NONE',  #7612 ) ;
#4947=VECTOR ( 'NONE', #2646, 1000.000000000000000 ) ;
#4948=ORIENTED_EDGE ( 'NONE', *, *, #6929, .F. ) ;
#4951=VECTOR ( 'NONE', #2261, 1000.000000000000000 ) ;
#4952=FACE_BOUND ( 'NONE', #593, .T. ) ;
#4961=LINE ( 'NONE', #4313, #2917 ) ;
#4963=DIRECTION ( 'NONE',  ( 0.000000000000000000, -0.000000000000000000, -1.000000000000000000 ) ) ;
#4974=AXIS2_PLACEMENT_3D ( 'NONE', #4507, #7587, #3287 ) ;
#4980=CIRCLE ( 'NONE', #1352, 5.999999999999991118 ) ;
#4984=ORIENTED_EDGE ( 'NONE', *, *, #6588, .F. ) ;
#4992=ORIENTED_EDGE ( 'NONE', *, *, #7798, .F. ) ;
#5005=LINE ( 'NONE', #3738, #8048 ) ;
#5021=CARTESIAN_POINT ( 'NONE',  ( -114.9999999999999147, -100.0000000000000000, 0.000000000000000000 ) ) ;
#5036=EDGE_CURVE ( 'NONE', #3000, #900, #1236, .T. ) ;
#5039=PLANE ( 'NONE',  #2560 ) ;
#5040=ADVANCED_FACE ( 'NONE', ( #4459 ), #1531, .T. ) ;
#5041=FACE_OUTER_BOUND ( 'NONE', #5112, .T. ) ;
#5045=DIRECTION ( 'NONE',  ( 0.000000000000000000, 0.000000000000000000, 1.000000000000000000 ) ) ;
#5065=AXIS2_PLACEMENT_3D ( 'NONE', #535, #5849, #659 ) ;
#5070=DIRECTION ( 'NONE',  ( -1.000000000000000000, 0.000000000000000000, 0.000000000000000000 ) ) ;
#5073=DIRECTION ( 'NONE',  ( 0.000000000000000000, 0.000000000000000000, -1.000000000000000000 ) ) ;
#5088=ORIENTED_EDGE ( 'NONE', *, *, #3950, .T. ) ;
#5091=CARTESIAN_POINT ( 'NONE',  ( 99.99999999999991473, -115.0000000000000000, 250.0000000000000000 ) ) ;
#5097=AXIS2_PLACEMENT_3D ( 'NONE', #3623, #4854, #2995 ) ;
#5099=ADVANCED_FACE ( 'NONE', ( #5188 ), #7782, .T. ) ;
#5104=CARTESIAN_POINT ( 'NONE',  ( 108.9999999999999147, -115.0000000000000000, 0.000000000000000000 ) ) ;
#5107=FACE_OUTER_BOUND ( 'NONE', #4812, .T. ) ;
#5111=DIRECTION ( 'NONE',  ( 1.000000000000000000, 0.000000000000000000, 0.000000000000000000 ) ) ;
#5112=EDGE_LOOP ( 'NONE', ( #4992, #3557, #4909, #4842 ) ) ;
#5113=DIRECTION ( 'NONE',  ( -0.000000000000000000, -0.000000000000000000, 1.000000000000000000 ) ) ;
#5114=CARTESIAN_POINT ( 'NONE',  ( 0.000000000000000000, -4.500000000000000000, -28.00000000000002487 ) ) ;
#5115=DIRECTION ( 'NONE',  ( -0.000000000000000000, 0.000000000000000000, 1.000000000000000000 ) ) ;
#5132=CARTESIAN_POINT ( 'NONE',  ( 114.9999999999999147, -100.0000000000000000, 0.000000000000000000 ) ) ;
#5135=DIRECTION ( 'NONE',  ( -0.000000000000000000, -0.000000000000000000, -1.000000000000000000 ) ) ;
#5159=EDGE_CURVE ( 'NONE', #471, #3015, #2813, .T. ) ;
#5164=VERTEX_POINT ( 'NONE', #5234 ) ;
#5169=FACE_OUTER_BOUND ( 'NONE', #7025, .T. ) ;
#5178=DIRECTION ( 'NONE',  ( -0.000000000000000000, -0.000000000000000000, 1.000000000000000000 ) ) ;
#5180=DIRECTION ( 'NONE',  ( 1.000000000000000000, 0.000000000000000000, 0.000000000000000000 ) ) ;
#5181=DIRECTION ( 'NONE',  ( -0.000000000000000000, -0.000000000000000000, 1.000000000000000000 ) ) ;
#5188=FACE_OUTER_BOUND ( 'NONE', #6843, .T. ) ;
#5194=CYLINDRICAL_SURFACE ( 'NONE', #6038, 5.000000000000004441 ) ;
#5200=DIRECTION ( 'NONE',  ( 0.000000000000000000, 0.000000000000000000, -1.000000000000000000 ) ) ;
#5205=EDGE_LOOP ( 'NONE', ( #3894, #6954 ) ) ;
#5220=VECTOR ( 'NONE', #450, 1000.000000000000000 ) ;
#5222=EDGE_LOOP ( 'NONE', ( #8166, #6764, #5619, #6255, #2557 ) ) ;
#5226=ORIENTED_EDGE ( 'NONE', *, *, #6227, .F. ) ;
#5231=DIRECTION ( 'NONE',  ( -0.000000000000000000, -0.000000000000000000, 1.000000000000000000 ) ) ;
#5233=VERTEX_POINT ( 'NONE', #4035 ) ;
#5234=CARTESIAN_POINT ( 'NONE',  ( -125.0000000000000000, 120.0000000000000000, -28.00000000000002487 ) ) ;
#5235=VECTOR ( 'NONE', #3526, 1000.000000000000000 ) ;
#5241=AXIS2_PLACEMENT_3D ( 'NONE', #2805, #7968, #6618 ) ;
#5247=AXIS2_PLACEMENT_3D ( 'NONE', #2562, #7725, #2446 ) ;
#5248=VECTOR ( 'NONE', #5135, 1000.000000000000000 ) ;
#5260=EDGE_CURVE ( 'NONE', #5164, #381, #105, .T. ) ;
#5261=EDGE_CURVE ( 'NONE', #1962, #6239, #2930, .T. ) ;
#5265=CARTESIAN_POINT ( 'NONE',  ( 99.99999999999990052, 115.0000000000000000, 250.0000000000000000 ) ) ;
#5269=ORIENTED_EDGE ( 'NONE', *, *, #1273, .T. ) ;
#5270=DIRECTION ( 'NONE',  ( -0.000000000000000000, -0.000000000000000000, -1.000000000000000000 ) ) ;
#5272=DIRECTION ( 'NONE',  ( -0.000000000000000000, -0.000000000000000000, 1.000000000000000000 ) ) ;
#5274=EDGE_CURVE ( 'NONE', #6076, #2040, #2660, .T. ) ;
#5276=CARTESIAN_POINT ( 'NONE',  ( 17.61817604250836311, 4.500000000000000000, -126.0000000000000284 ) ) ;
#5309=VERTEX_POINT ( 'NONE', #926 ) ;
#5315=VERTEX_POINT ( 'NONE', #2935 ) ;
#5329=EDGE_LOOP ( 'NONE', ( #4860, #6097, #2996, #668 ) ) ;
#5330=LINE ( 'NONE', #857, #6413 ) ;
#5332=CARTESIAN_POINT ( 'NONE',  ( 15.00000000000000000, 0.000000000000000000, -128.0000000000000284 ) ) ;
#5334=CARTESIAN_POINT ( 'NONE',  ( 0.000000000000000000, -15.00000000000000000, -126.0000000000000284 ) ) ;
#5336=CIRCLE ( 'NONE', #4516, 5.999999999999991118 ) ;
#5340=CARTESIAN_POINT ( 'NONE',  ( 17.61817604250836311, 4.500000000000000000, -128.0000000000000284 ) ) ;
#5350=ORIENTED_EDGE ( 'NONE', *, *, #2640, .F. ) ;
#5356=AXIS2_PLACEMENT_3D ( 'NONE', #2240, #5383, #869 ) ;
#5363=DIRECTION ( 'NONE',  ( 0.000000000000000000, -0.000000000000000000, -1.000000000000000000 ) ) ;
#5376=FACE_OUTER_BOUND ( 'NONE', #1013, .T. ) ;
#5383=DIRECTION ( 'NONE',  ( -0.000000000000000000, 0.000000000000000000, 1.000000000000000000 ) ) ;
#5389=VERTEX_POINT ( 'NONE', #6142 ) ;
#5390=DIRECTION ( 'NONE',  ( -1.000000000000000000, 0.000000000000000000, 0.000000000000000000 ) ) ;
#5404=EDGE_CURVE ( 'NONE', #4206, #8026, #2364, .T. ) ;
#5410=CARTESIAN_POINT ( 'NONE',  ( -120.9999999999999005, -115.0000000000000000, 0.000000000000000000 ) ) ;
#5413=VECTOR ( 'NONE', #7779, 1000.000000000000000 ) ;
#5455=ADVANCED_FACE ( 'NONE', ( #1298 ), #7080, .F. ) ;
#5459=DIRECTION ( 'NONE',  ( 1.000000000000000000, 0.000000000000000000, 0.000000000000000000 ) ) ;
#5464=DIRECTION ( 'NONE',  ( 0.000000000000000000, -1.000000000000000000, 0.000000000000000000 ) ) ;
#5469=CARTESIAN_POINT ( 'NONE',  ( 0.000000000000000000, -4.500000000000000000, -128.0000000000000284 ) ) ;
#5475=EDGE_CURVE ( 'NONE', #4379, #6239, #7597, .T. ) ;
#5480=VERTEX_POINT ( 'NONE', #1818 ) ;
#5483=ORIENTED_EDGE ( 'NONE', *, *, #3439, .T. ) ;
#5496=ORIENTED_EDGE ( 'NONE', *, *, #198, .T. ) ;
#5502=CARTESIAN_POINT ( 'NONE',  ( 0.000000000000000000, 0.000000000000000000, -128.0000000000000284 ) ) ;
#5503=ADVANCED_FACE ( 'NONE', ( #3744 ), #3228, .F. ) ;
#5510=VERTEX_POINT ( 'NONE', #7040 ) ;
#5513=CYLINDRICAL_SURFACE ( 'NONE', #350, 5.999999999999991118 ) ;
#5520=CIRCLE ( 'NONE', #383, 15.00000000000000000 ) ;
#5535=DIRECTION ( 'NONE',  ( 0.000000000000000000, 1.000000000000000000, -0.000000000000000000 ) ) ;
#5536=PRODUCT_DEFINITION_SHAPE ( 'NONE', 'NONE',  #7576 ) ;
#5538=CARTESIAN_POINT ( 'NONE',  ( -108.9999999999999147, -115.0000000000000000, 0.000000000000000000 ) ) ;
#5541=VERTEX_POINT ( 'NONE', #3830 ) ;
#5544=ORIENTED_EDGE ( 'NONE', *, *, #4523, .T. ) ;
#5553=LINE ( 'NONE', #3102, #3865 ) ;
#5570=DIRECTION ( 'NONE',  ( 0.000000000000000000, 1.000000000000000000, -0.000000000000000000 ) ) ;
#5577=LINE ( 'NONE', #8021, #5235 ) ;
#5578=ORIENTED_EDGE ( 'NONE', *, *, #1026, .T. ) ;
#5584=VERTEX_POINT ( 'NONE', #5091 ) ;
#5585=EDGE_CURVE ( 'NONE', #2918, #6076, #6997, .T. ) ;
#5587=CARTESIAN_POINT ( 'NONE',  ( -125.0000000000000000, -125.0000000000000000, -28.00000000000002487 ) ) ;
#5600=CARTESIAN_POINT ( 'NONE',  ( -114.9999999999999147, -115.0000000000000000, 0.000000000000000000 ) ) ;
#5607=EDGE_CURVE ( 'NONE', #1156, #1010, #6268, .T. ) ;
#5615=AXIS2_PLACEMENT_3D ( 'NONE', #3785, #620, #5768 ) ;
#5616=VERTEX_POINT ( 'NONE', #6436 ) ;
#5617=DIRECTION ( 'NONE',  ( 0.000000000000000000, -0.000000000000000000, -1.000000000000000000 ) ) ;
#5619=ORIENTED_EDGE ( 'NONE', *, *, #4100, .F. ) ;
#5622=EDGE_CURVE ( 'NONE', #3739, #4104, #244, .T. ) ;
#5623=EDGE_CURVE ( 'NONE', #471, #8026, #141, .T. ) ;
#5625=AXIS2_PLACEMENT_3D ( 'NONE', #823, #4560, #1373 ) ;
#5628=CARTESIAN_POINT ( 'NONE',  ( -99.99999999999991473, -115.0000000000000000, 250.0000000000000000 ) ) ;
#5632=CARTESIAN_POINT ( 'NONE',  ( 14.30908802125418511, -4.500000000000000000, -118.0000000000000284 ) ) ;
#5643=EDGE_LOOP ( 'NONE', ( #3634, #2651, #8183, #5496 ) ) ;
#5650=CARTESIAN_POINT ( 'NONE',  ( 0.000000000000000000, 115.0000000000000000, 250.0000000000000000 ) ) ;
#5653=AXIS2_PLACEMENT_3D ( 'NONE', #3699, #5815, #1264 ) ;
#5659=DIRECTION ( 'NONE',  ( -1.000000000000000000, 0.000000000000000000, 0.000000000000000000 ) ) ;
#5680=FACE_OUTER_BOUND ( 'NONE', #6190, .T. ) ;
#5682=FACE_OUTER_BOUND ( 'NONE', #1100, .T. ) ;
#5685=CARTESIAN_POINT ( 'NONE',  ( 114.9999999999999147, 0.000000000000000000, 250.0000000000000000 ) ) ;
#5690=ORIENTED_EDGE ( 'NONE', *, *, #3764, .F. ) ;
#5693=ORIENTED_EDGE ( 'NONE', *, *, #3628, .T. ) ;
#5707=CARTESIAN_POINT ( 'NONE',  ( 0.000000000000000000, 0.000000000000000000, -120.5000000000000284 ) ) ;
#5712=DIRECTION ( 'NONE',  ( -0.000000000000000000, 0.000000000000000000, 1.000000000000000000 ) ) ;
#5719=CARTESIAN_POINT ( 'NONE',  ( 0.000000000000000000, 0.000000000000000000, -126.0000000000000284 ) ) ;
#5722=ADVANCED_FACE ( 'NONE', ( #181 ), #2759, .F. ) ;
#5744=LINE ( 'NONE', #1563, #4289 ) ;
#5763=DIRECTION ( 'NONE',  ( -0.000000000000000000, -0.000000000000000000, -1.000000000000000000 ) ) ;
#5768=DIRECTION ( 'NONE',  ( 0.000000000000000000, 0.000000000000000000, -1.000000000000000000 ) ) ;
#5769=AXIS2_PLACEMENT_3D ( 'NONE', #5685, #6390, #5045 ) ;
#5780=DIRECTION ( 'NONE',  ( -0.000000000000000000, -0.000000000000000000, -1.000000000000000000 ) ) ;
#5806=ORIENTED_EDGE ( 'NONE', *, *, #2238, .F. ) ;
#5815=DIRECTION ( 'NONE',  ( -0.000000000000000000, -0.000000000000000000, 1.000000000000000000 ) ) ;
#5833=LINE ( 'NONE', #6342, #7526 ) ;
#5835=FACE_BOUND ( 'NONE', #7259, .T. ) ;
#5838=CARTESIAN_POINT ( 'NONE',  ( 14.30908802125418511, -4.500000000000000000, -126.0000000000000284 ) ) ;
#5839=ORIENTED_EDGE ( 'NONE', *, *, #7163, .T. ) ;
#5840=ADVANCED_FACE ( 'NONE', ( #7965 ), #3550, .T. ) ;
#5841=CARTESIAN_POINT ( 'NONE',  ( -120.0000000000000000, -120.0000000000000000, -28.00000000000002487 ) ) ;
#5849=DIRECTION ( 'NONE',  ( 0.000000000000000000, 0.000000000000000000, -1.000000000000000000 ) ) ;
#5851=ORIENTED_EDGE ( 'NONE', *, *, #4417, .T. ) ;
#5862=ORIENTED_EDGE ( 'NONE', *, *, #615, .T. ) ;
#5884=CARTESIAN_POINT ( 'NONE',  ( 0.000000000000000000, 0.000000000000000000, 0.000000000000000000 ) ) ;
#5900=AXIS2_PLACEMENT_3D ( 'NONE', #4716, #70, #2210 ) ;
#5911=DIRECTION ( 'NONE',  ( -1.000000000000000000, 0.000000000000000000, 0.000000000000000000 ) ) ;
#5916=CARTESIAN_POINT ( 'NONE',  ( -120.0000000000000000, 125.0000000000000000, -28.00000000000002487 ) ) ;
#5922=CIRCLE ( 'NONE', #3219, 15.00000000000001421 ) ;
#5925=LINE ( 'NONE', #1659, #1446 ) ;
#5927=DIRECTION ( 'NONE',  ( 1.000000000000000000, 0.000000000000000000, 0.000000000000000000 ) ) ;
#5928=EDGE_CURVE ( 'NONE', #5510, #1156, #2433, .T. ) ;
#5931=AXIS2_PLACEMENT_3D ( 'NONE', #4847, #4196, #7437 ) ;
#5933=ORIENTED_EDGE ( 'NONE', *, *, #7029, .F. ) ;
#5934=DIRECTION ( 'NONE',  ( -0.000000000000000000, -0.000000000000000000, 1.000000000000000000 ) ) ;
#5939=DIRECTION ( 'NONE',  ( 0.000000000000000000, -0.000000000000000000, -1.000000000000000000 ) ) ;
#5941=ADVANCED_FACE ( 'NONE', ( #4952, #7628, #2482, #1128, #5835, #3733 ), #5039, .F. ) ;
#5942=CARTESIAN_POINT ( 'NONE',  ( -114.9999999999999147, 115.0000000000000000, 8.205133554287239938E-16 ) ) ;
#5953=LINE ( 'NONE', #4681, #229 ) ;
#5955=CARTESIAN_POINT ( 'NONE',  ( -114.9999999999999147, 115.0000000000000000, 250.0000000000000000 ) ) ;
#5960=ORIENTED_EDGE ( 'NONE', *, *, #2585, .T. ) ;
#5969=CARTESIAN_POINT ( 'NONE',  ( 125.0000000000000000, -120.0000000000000000, -28.00000000000002487 ) ) ;
#5980=LINE ( 'NONE', #65, #7724 ) ;
#5984=ORIENTED_EDGE ( 'NONE', *, *, #6794, .T. ) ;
#5998=CYLINDRICAL_SURFACE ( 'NONE', #2519, 14.99999999999998579 ) ;
#6007=ORIENTED_EDGE ( 'NONE', *, *, #4204, .T. ) ;
#6025=CIRCLE ( 'NONE', #7810, 15.00000000000000000 ) ;
#6027=DIRECTION ( 'NONE',  ( -0.000000000000000000, -0.000000000000000000, 1.000000000000000000 ) ) ;
#6035=DIRECTION ( 'NONE',  ( -0.000000000000000000, -0.000000000000000000, 1.000000000000000000 ) ) ;
#6038=AXIS2_PLACEMENT_3D ( 'NONE', #2170, #7139, #1364 ) ;
#6043=CARTESIAN_POINT ( 'NONE',  ( -99.99999999999990052, 115.0000000000000000, 250.0000000000000000 ) ) ;
#6044=FACE_OUTER_BOUND ( 'NONE', #755, .T. ) ;
#6056=LINE ( 'NONE', #271, #185 ) ;
#6058=ORIENTED_EDGE ( 'NONE', *, *, #7323, .F. ) ;
#6066=ORIENTED_EDGE ( 'NONE', *, *, #7581, .F. ) ;
#6067=CARTESIAN_POINT ( 'NONE',  ( 99.99999999999990052, 115.0000000000000000, 0.000000000000000000 ) ) ;
#6076=VERTEX_POINT ( 'NONE', #4726 ) ;
#6085=CARTESIAN_POINT ( 'NONE',  ( 17.61817604250836311, -4.500000000000000000, -120.5000000000000284 ) ) ;
#6088=CARTESIAN_POINT ( 'NONE',  ( 0.000000000000000000, 0.000000000000000000, -126.0000000000000284 ) ) ;
#6090=CYLINDRICAL_SURFACE ( 'NONE', #6455, 15.00000000000000000 ) ;
#6096=CARTESIAN_POINT ( 'NONE',  ( 14.30908802125418511, 4.500000000000000000, -128.0000000000000284 ) ) ;
#6097=ORIENTED_EDGE ( 'NONE', *, *, #6105, .T. ) ;
#6105=EDGE_CURVE ( 'NONE', #5480, #902, #2104, .T. ) ;
#6106=CIRCLE ( 'NONE', #6792, 15.00000000000000000 ) ;
#6110=ORIENTED_EDGE ( 'NONE', *, *, #7581, .T. ) ;
#6114=ADVANCED_FACE ( 'NONE', ( #3365 ), #4126, .F. ) ;
#6115=ORIENTED_EDGE ( 'NONE', *, *, #5159, .F. ) ;
#6117=CARTESIAN_POINT ( 'NONE',  ( 114.9999999999999147, -115.0000000000000000, 0.000000000000000000 ) ) ;
#6120=( NAMED_UNIT ( * ) PLANE_ANGLE_UNIT ( ) SI_UNIT ( $, .RADIAN. ) );
#6124=VERTEX_POINT ( 'NONE', #7871 ) ;
#6128=DIRECTION ( 'NONE',  ( 0.000000000000000000, -0.000000000000000000, -1.000000000000000000 ) ) ;
#6129=AXIS2_PLACEMENT_3D ( 'NONE', #6160, #7527, #380 ) ;
#6132=CARTESIAN_POINT ( 'NONE',  ( -114.9999999999999147, 99.99999999999998579, 250.0000000000000000 ) ) ;
#6139=AXIS2_PLACEMENT_3D ( 'NONE', #2108, #3369, #4649 ) ;
#6142=CARTESIAN_POINT ( 'NONE',  ( -99.99999999999991473, -115.0000000000000000, 250.0000000000000000 ) ) ;
#6152=VECTOR ( 'NONE', #4210, 1000.000000000000000 ) ;
#6157=ORIENTED_EDGE ( 'NONE', *, *, #7602, .F. ) ;
#6160=CARTESIAN_POINT ( 'NONE',  ( 120.0000000000000000, 120.0000000000000000, -28.00000000000002487 ) ) ;
#6164=FACE_OUTER_BOUND ( 'NONE', #3149, .T. ) ;
#6166=CYLINDRICAL_SURFACE ( 'NONE', #3772, 5.999999999999991118 ) ;
#6173=ORIENTED_EDGE ( 'NONE', *, *, #2828, .F. ) ;
#6177=CARTESIAN_POINT ( 'NONE',  ( 114.9999999999999147, -115.0000000000000000, 0.000000000000000000 ) ) ;
#6180=DIRECTION ( 'NONE',  ( 1.000000000000000000, 0.000000000000000000, 0.000000000000000000 ) ) ;
#6190=EDGE_LOOP ( 'NONE', ( #3788, #7191, #6535, #4409, #8171, #3493, #6910, #2639 ) ) ;
#6194=ADVANCED_FACE ( 'NONE', ( #7354 ), #1573, .T. ) ;
#6195=FACE_OUTER_BOUND ( 'NONE', #1728, .T. ) ;
#6207=ORIENTED_EDGE ( 'NONE', *, *, #1273, .F. ) ;
#6215=VERTEX_POINT ( 'NONE', #7569 ) ;
#6219=CARTESIAN_POINT ( 'NONE',  ( 0.000000000000000000, 0.000000000000000000, -28.00000000000002487 ) ) ;
#6227=EDGE_CURVE ( 'NONE', #6430, #1402, #331, .T. ) ;
#6232=CARTESIAN_POINT ( 'NONE',  ( 0.000000000000000000, -4.500000000000000000, -126.0000000000000284 ) ) ;
#6239=VERTEX_POINT ( 'NONE', #2900 ) ;
#6244=DIRECTION ( 'NONE',  ( 1.000000000000000000, 0.000000000000000000, 0.000000000000000000 ) ) ;
#6246=VERTEX_POINT ( 'NONE', #6286 ) ;
#6251=DIRECTION ( 'NONE',  ( -0.000000000000000000, -0.000000000000000000, 1.000000000000000000 ) ) ;
#6255=ORIENTED_EDGE ( 'NONE', *, *, #581, .F. ) ;
#6257=ORIENTED_EDGE ( 'NONE', *, *, #1046, .T. ) ;
#6265=ORIENTED_EDGE ( 'NONE', *, *, #1745, .F. ) ;
#6268=LINE ( 'NONE', #2573, #5248 ) ;
#6274=CARTESIAN_POINT ( 'NONE',  ( -125.0000000000000000, -125.0000000000000000, -28.00000000000002487 ) ) ;
#6275=EDGE_CURVE ( 'NONE', #7952, #698, #6998, .T. ) ;
#6283=DIRECTION ( 'NONE',  ( -0.000000000000000000, -0.000000000000000000, 1.000000000000000000 ) ) ;
#6286=CARTESIAN_POINT ( 'NONE',  ( 114.9999999999999147, 99.99999999999998579, 0.000000000000000000 ) ) ;
#6287=CARTESIAN_POINT ( 'NONE',  ( 108.9999999999999147, -115.0000000000000000, -28.00000000000002487 ) ) ;
#6288=AXIS2_PLACEMENT_3D ( 'NONE', #6219, #2354, #347 ) ;
#6289=ADVANCED_FACE ( 'NONE', ( #4895 ), #3082, .F. ) ;
#6293=CIRCLE ( 'NONE', #4939, 5.999999999999991118 ) ;
#6296=AXIS2_PLACEMENT_3D ( 'NONE', #3692, #8228, #2362 ) ;
#6305=AXIS2_PLACEMENT_3D ( 'NONE', #7792, #2016, #122 ) ;
#6311=CARTESIAN_POINT ( 'NONE',  ( 0.000000000000000000, 0.000000000000000000, 0.000000000000000000 ) ) ;
#6316=AXIS2_PLACEMENT_3D ( 'NONE', #2292, #3517, #1011 ) ;
#6321=VERTEX_POINT ( 'NONE', #8153 ) ;
#6342=CARTESIAN_POINT ( 'NONE',  ( -125.0000000000000000, -125.0000000000000000, -28.00000000000002487 ) ) ;
#6356=ORIENTED_EDGE ( 'NONE', *, *, #4633, .T. ) ;
#6374=DIRECTION ( 'NONE',  ( 1.000000000000000000, 0.000000000000000000, 0.000000000000000000 ) ) ;
#6383=ADVANCED_FACE ( 'NONE', ( #5107 ), #7701, .F. ) ;
#6390=DIRECTION ( 'NONE',  ( -1.000000000000000000, 0.000000000000000000, 0.000000000000000000 ) ) ;
#6391=VECTOR ( 'NONE', #7298, 1000.000000000000000 ) ;
#6401=VERTEX_POINT ( 'NONE', #3161 ) ;
#6413=VECTOR ( 'NONE', #83, 1000.000000000000000 ) ;
#6414=DIRECTION ( 'NONE',  ( -1.000000000000000000, 0.000000000000000000, 0.000000000000000000 ) ) ;
#6421=DIRECTION ( 'NONE',  ( -0.000000000000000000, -0.000000000000000000, -1.000000000000000000 ) ) ;
#6430=VERTEX_POINT ( 'NONE', #1196 ) ;
#6434=EDGE_CURVE ( 'NONE', #5584, #5389, #5744, .T. ) ;
#6435=ORIENTED_EDGE ( 'NONE', *, *, #6866, .F. ) ;
#6436=CARTESIAN_POINT ( 'NONE',  ( -108.9999999999999147, -115.0000000000000000, -28.00000000000002487 ) ) ;
#6445=CARTESIAN_POINT ( 'NONE',  ( 14.30908802125418511, -4.500000000000000000, -118.0000000000000284 ) ) ;
#6446=ORIENTED_EDGE ( 'NONE', *, *, #5404, .F. ) ;
#6455=AXIS2_PLACEMENT_3D ( 'NONE', #315, #3596, #6180 ) ;
#6458=EDGE_LOOP ( 'NONE', ( #3417, #1153, #1978, #5984 ) ) ;
#6460=DIRECTION ( 'NONE',  ( -1.000000000000000000, 0.000000000000000000, 0.000000000000000000 ) ) ;
#6464=CARTESIAN_POINT ( 'NONE',  ( 120.0000000000000000, -120.0000000000000000, -28.00000000000002487 ) ) ;
#6481=DIRECTION ( 'NONE',  ( 1.000000000000000000, 0.000000000000000000, 0.000000000000000000 ) ) ;
#6486=AXIS2_PLACEMENT_3D ( 'NONE', #5942, #5231, #3308 ) ;
#6503=LINE ( 'NONE', #4601, #8008 ) ;
#6522=LINE ( 'NONE', #7849, #7384 ) ;
#6525=VERTEX_POINT ( 'NONE', #1479 ) ;
#6527=ORIENTED_EDGE ( 'NONE', *, *, #1990, .T. ) ;
#6528=LINE ( 'NONE', #751, #8066 ) ;
#6535=ORIENTED_EDGE ( 'NONE', *, *, #5274, .F. ) ;
#6541=DIRECTION ( 'NONE',  ( 0.000000000000000000, 0.000000000000000000, -1.000000000000000000 ) ) ;
#6543=EDGE_LOOP ( 'NONE', ( #8032, #2445, #515, #1510 ) ) ;
#6547=EDGE_CURVE ( 'NONE', #6215, #6401, #7976, .T. ) ;
#6568=FACE_OUTER_BOUND ( 'NONE', #5329, .T. ) ;
#6573=DIRECTION ( 'NONE',  ( 0.000000000000000000, -0.000000000000000000, -1.000000000000000000 ) ) ;
#6584=DIRECTION ( 'NONE',  ( -0.000000000000000000, -0.000000000000000000, -1.000000000000000000 ) ) ;
#6588=EDGE_CURVE ( 'NONE', #7585, #3267, #243, .T. ) ;
#6601=EDGE_CURVE ( 'NONE', #4386, #4206, #4697, .T. ) ;
#6607=CYLINDRICAL_SURFACE ( 'NONE', #1550, 25.00000000000000000 ) ;
#6618=DIRECTION ( 'NONE',  ( -1.000000000000000000, 0.000000000000000000, 0.000000000000000000 ) ) ;
#6620=DIRECTION ( 'NONE',  ( -0.000000000000000000, -0.000000000000000000, -1.000000000000000000 ) ) ;
#6626=ADVANCED_BREP_SHAPE_REPRESENTATION ( '', ( #706, #1299 ), #7463 ) ;
#6630=DIRECTION ( 'NONE',  ( -0.000000000000000000, 0.000000000000000000, -1.000000000000000000 ) ) ;
#6654=DIRECTION ( 'NONE',  ( -1.000000000000000000, 0.000000000000000000, 0.000000000000000000 ) ) ;
#6663=DIRECTION ( 'NONE',  ( -1.000000000000000000, 0.000000000000000000, 0.000000000000000000 ) ) ;
#6667=ADVANCED_FACE ( 'NONE', ( #2412 ), #7434, .T. ) ;
#6678=DIRECTION ( 'NONE',  ( 0.000000000000000000, 1.000000000000000000, 0.000000000000000000 ) ) ;
#6681=DIRECTION ( 'NONE',  ( -0.000000000000000000, -0.000000000000000000, 1.000000000000000000 ) ) ;
#6683=CARTESIAN_POINT ( 'NONE',  ( -114.9999999999999147, -115.0000000000000000, 250.0000000000000000 ) ) ;
#6685=DIRECTION ( 'NONE',  ( -0.000000000000000000, 0.000000000000000000, 1.000000000000000000 ) ) ;
#6703=CARTESIAN_POINT ( 'NONE',  ( 14.30908802125418511, 4.500000000000000000, -118.0000000000000284 ) ) ;
#6714=CARTESIAN_POINT ( 'NONE',  ( -114.9999999999999147, 0.000000000000000000, 250.0000000000000000 ) ) ;
#6726=CARTESIAN_POINT ( 'NONE',  ( 17.61817604250836311, 4.500000000000000000, -128.0000120000000265 ) ) ;
#6729=VECTOR ( 'NONE', #2483, 1000.000000000000000 ) ;
#6736=EDGE_LOOP ( 'NONE', ( #3908, #2688, #1963, #2726 ) ) ;
#6738=ORIENTED_EDGE ( 'NONE', *, *, #3693, .T. ) ;
#6745=UNCERTAINTY_MEASURE_WITH_UNIT (LENGTH_MEASURE( 1.000000000000000082E-05 ), #2929, 'distance_accuracy_value', 'NONE');
#6753=ORIENTED_EDGE ( 'NONE', *, *, #1938, .T. ) ;
#6763=DIRECTION ( 'NONE',  ( -0.000000000000000000, -0.000000000000000000, 1.000000000000000000 ) ) ;
#6764=ORIENTED_EDGE ( 'NONE', *, *, #6917, .T. ) ;
#6765=EDGE_CURVE ( 'NONE', #1962, #471, #7642, .T. ) ;
#6767=CARTESIAN_POINT ( 'NONE',  ( -114.9999999999999147, -115.0000000000000000, 8.205133554287239938E-16 ) ) ;
#6782=ORIENTED_EDGE ( 'NONE', *, *, #4837, .T. ) ;
#6783=CARTESIAN_POINT ( 'NONE',  ( 0.000000000000000000, -4.500000000000000000, -128.0000120000000265 ) ) ;
#6789=CARTESIAN_POINT ( 'NONE',  ( -114.9999999999999147, 0.000000000000000000, 0.000000000000000000 ) ) ;
#6791=EDGE_CURVE ( 'NONE', #5584, #1787, #7001, .T. ) ;
#6792=AXIS2_PLACEMENT_3D ( 'NONE', #6088, #8222, #1767 ) ;
#6793=CARTESIAN_POINT ( 'NONE',  ( -99.99999999999991473, -115.0000000000000000, 0.000000000000000000 ) ) ;
#6794=EDGE_CURVE ( 'NONE', #4868, #8098, #589, .T. ) ;
#6843=EDGE_LOOP ( 'NONE', ( #687, #7641, #7574, #6066 ) ) ;
#6858=VECTOR ( 'NONE', #1224, 1000.000000000000000 ) ;
#6866=EDGE_CURVE ( 'NONE', #5233, #2019, #2807, .T. ) ;
#6868=VERTEX_POINT ( 'NONE', #183 ) ;
#6873=ORIENTED_EDGE ( 'NONE', *, *, #2616, .T. ) ;
#6879=ORIENTED_EDGE ( 'NONE', *, *, #7662, .F. ) ;
#6893=CARTESIAN_POINT ( 'NONE',  ( 0.000000000000000000, -15.00000000000000000, -120.5000000000000284 ) ) ;
#6906=CARTESIAN_POINT ( 'NONE',  ( 120.0000000000000000, -120.0000000000000000, -28.00000000000002487 ) ) ;
#6910=ORIENTED_EDGE ( 'NONE', *, *, #4651, .T. ) ;
#6917=EDGE_CURVE ( 'NONE', #2291, #6401, #2729, .T. ) ;
#6918=CARTESIAN_POINT ( 'NONE',  ( 114.9999999999999147, 115.0000000000000000, 8.205133554287239938E-16 ) ) ;
#6929=EDGE_CURVE ( 'NONE', #6868, #4386, #6528, .T. ) ;
#6931=ORIENTED_EDGE ( 'NONE', *, *, #3133, .F. ) ;
#6933=CARTESIAN_POINT ( 'NONE',  ( 114.9999999999999147, 115.0000000000000000, -28.00000000000002487 ) ) ;
#6937=EDGE_LOOP ( 'NONE', ( #1018, #2596, #3502, #7525 ) ) ;
#6940=DIRECTION ( 'NONE',  ( 1.000000000000000000, 0.000000000000000000, 0.000000000000000000 ) ) ;
#6942=ORIENTED_EDGE ( 'NONE', *, *, #1988, .F. ) ;
#6944=DIRECTION ( 'NONE',  ( 1.000000000000000000, 0.000000000000000000, 0.000000000000000000 ) ) ;
#6952=EDGE_CURVE ( 'NONE', #5584, #6430, #3891, .T. ) ;
#6954=ORIENTED_EDGE ( 'NONE', *, *, #3961, .T. ) ;
#6961=SHAPE_DEFINITION_REPRESENTATION ( #5536, #1440 ) ;
#6963=EDGE_LOOP ( 'NONE', ( #4782, #6115, #4489, #960 ) ) ;
#6970=ORIENTED_EDGE ( 'NONE', *, *, #295, .T. ) ;
#6974=ORIENTED_EDGE ( 'NONE', *, *, #973, .F. ) ;
#6984=ORIENTED_EDGE ( 'NONE', *, *, #5928, .T. ) ;
#6997=LINE ( 'NONE', #5969, #108 ) ;
#6998=CIRCLE ( 'NONE', #3342, 5.000000000000004441 ) ;
#7001=LINE ( 'NONE', #3150, #2289 ) ;
#7019=ORIENTED_EDGE ( 'NONE', *, *, #4381, .T. ) ;
#7020=DIRECTION ( 'NONE',  ( 1.000000000000000000, 0.000000000000000000, 0.000000000000000000 ) ) ;
#7025=EDGE_LOOP ( 'NONE', ( #4175, #3039, #3881, #4889 ) ) ;
#7027=AXIS2_PLACEMENT_3D ( 'NONE', #3026, #7046, #5659 ) ;
#7029=EDGE_CURVE ( 'NONE', #306, #3000, #3341, .T. ) ;
#7032=DIRECTION ( 'NONE',  ( -0.000000000000000000, 0.000000000000000000, 1.000000000000000000 ) ) ;
#7038=ORIENTED_EDGE ( 'NONE', *, *, #1285, .F. ) ;
#7040=CARTESIAN_POINT ( 'NONE',  ( 25.00000000000000000, 3.061616997868383043E-15, -120.5000000000000284 ) ) ;
#7041=ORIENTED_EDGE ( 'NONE', *, *, #2835, .T. ) ;
#7043=CIRCLE ( 'NONE', #1795, 5.000000000000004441 ) ;
#7046=DIRECTION ( 'NONE',  ( 0.000000000000000000, 0.000000000000000000, -1.000000000000000000 ) ) ;
#7054=CARTESIAN_POINT ( 'NONE',  ( -25.00000000000000000, 0.000000000000000000, -126.0000000000000284 ) ) ;
#7057=CARTESIAN_POINT ( 'NONE',  ( -114.9999999999999147, -115.0000000000000000, 8.205133554287239938E-16 ) ) ;
#7066=ADVANCED_FACE ( 'NONE', ( #4222 ), #6090, .T. ) ;
#7069=PLANE ( 'NONE',  #4355 ) ;
#7080=PLANE ( 'NONE',  #377 ) ;
#7092=VECTOR ( 'NONE', #5111, 1000.000000000000000 ) ;
#7097=DIRECTION ( 'NONE',  ( -0.000000000000000000, -0.000000000000000000, 1.000000000000000000 ) ) ;
#7132=VECTOR ( 'NONE', #5180, 1000.000000000000000 ) ;
#7134=DIRECTION ( 'NONE',  ( 0.000000000000000000, 1.000000000000000000, 0.000000000000000000 ) ) ;
#7139=DIRECTION ( 'NONE',  ( 0.000000000000000000, 0.000000000000000000, -1.000000000000000000 ) ) ;
#7163=EDGE_CURVE ( 'NONE', #2019, #5164, #1845, .T. ) ;
#7164=CIRCLE ( 'NONE', #7027, 15.00000000000000000 ) ;
#7176=CARTESIAN_POINT ( 'NONE',  ( 0.000000000000000000, 0.000000000000000000, -126.0000000000000284 ) ) ;
#7178=ADVANCED_FACE ( 'NONE', ( #5682 ), #3687, .F. ) ;
#7184=EDGE_CURVE ( 'NONE', #5389, #6321, #5520, .T. ) ;
#7187=VERTEX_POINT ( 'NONE', #8224 ) ;
#7190=DIRECTION ( 'NONE',  ( 1.000000000000000000, 0.000000000000000000, 0.000000000000000000 ) ) ;
#7191=ORIENTED_EDGE ( 'NONE', *, *, #991, .T. ) ;
#7208=CARTESIAN_POINT ( 'NONE',  ( 114.9999999999999147, -115.0000000000000000, 0.000000000000000000 ) ) ;
#7213=ORIENTED_EDGE ( 'NONE', *, *, #4254, .T. ) ;
#7233=CARTESIAN_POINT ( 'NONE',  ( -15.00000000000000000, 1.836970198721029589E-15, -28.00000000000002487 ) ) ;
#7240=DIRECTION ( 'NONE',  ( -0.000000000000000000, -0.000000000000000000, 1.000000000000000000 ) ) ;
#7250=CARTESIAN_POINT ( 'NONE',  ( 114.9999999999999147, -115.0000000000000000, 250.0000000000000000 ) ) ;
#7255=EDGE_CURVE ( 'NONE', #7187, #7585, #1939, .T. ) ;
#7259=EDGE_LOOP ( 'NONE', ( #7038, #8113, #8027, #6931, #5483, #254, #5269, #6157 ) ) ;
#7261=CIRCLE ( 'NONE', #3887, 15.00000000000000000 ) ;
#7270=DIRECTION ( 'NONE',  ( -1.000000000000000000, 0.000000000000000000, 0.000000000000000000 ) ) ;
#7277=CARTESIAN_POINT ( 'NONE',  ( 114.9999999999999147, 0.000000000000000000, 250.0000000000000000 ) ) ;
#7281=VECTOR ( 'NONE', #3479, 1000.000000000000000 ) ;
#7298=DIRECTION ( 'NONE',  ( -0.000000000000000000, -0.000000000000000000, -1.000000000000000000 ) ) ;
#7320=DIRECTION ( 'NONE',  ( 1.000000000000000000, 0.000000000000000000, 0.000000000000000000 ) ) ;
#7323=EDGE_CURVE ( 'NONE', #6239, #3602, #802, .T. ) ;
#7328=DIRECTION ( 'NONE',  ( 1.000000000000000000, 0.000000000000000000, 0.000000000000000000 ) ) ;
#7354=FACE_OUTER_BOUND ( 'NONE', #2888, .T. ) ;
#7363=CARTESIAN_POINT ( 'NONE',  ( 0.000000000000000000, 0.000000000000000000, -128.0000000000000284 ) ) ;
#7364=DIRECTION ( 'NONE',  ( 0.000000000000000000, 0.000000000000000000, 1.000000000000000000 ) ) ;
#7384=VECTOR ( 'NONE', #3863, 1000.000000000000000 ) ;
#7395=DIRECTION ( 'NONE',  ( 0.000000000000000000, -1.000000000000000000, 0.000000000000000000 ) ) ;
#7396=CIRCLE ( 'NONE', #371, 5.999999999999991118 ) ;
#7422=CARTESIAN_POINT ( 'NONE',  ( 114.9999999999999147, -115.0000000000000000, -28.00000000000002487 ) ) ;
#7423=DIRECTION ( 'NONE',  ( -0.000000000000000000, -0.000000000000000000, 1.000000000000000000 ) ) ;
#7434=PLANE ( 'NONE',  #7940 ) ;
#7437=DIRECTION ( 'NONE',  ( 1.000000000000000000, 0.000000000000000000, 0.000000000000000000 ) ) ;
#7459=DIRECTION ( 'NONE',  ( -0.000000000000000000, -0.000000000000000000, 1.000000000000000000 ) ) ;
#7463=( GEOMETRIC_REPRESENTATION_CONTEXT ( 3 ) GLOBAL_UNCERTAINTY_ASSIGNED_CONTEXT ( ( #1855 ) ) GLOBAL_UNIT_ASSIGNED_CONTEXT ( ( #3540, #6120, #342 ) ) REPRESENTATION_CONTEXT ( 'NONE', 'WORKASPACE' ) );
#7468=ORIENTED_EDGE ( 'NONE', *, *, #5159, .T. ) ;
#7471=ADVANCED_FACE ( 'NONE', ( #2029 ), #6166, .F. ) ;
#7489=AXIS2_PLACEMENT_3D ( 'NONE', #6767, #7240, #831 ) ;
#7491=CARTESIAN_POINT ( 'NONE',  ( -114.9999999999999147, 99.99999999999998579, 250.0000000000000000 ) ) ;
#7509=DIRECTION ( 'NONE',  ( 1.000000000000000000, 0.000000000000000000, 0.000000000000000000 ) ) ;
#7511=PRODUCT_CONTEXT ( 'NONE', #7867, 'mechanical' ) ;
#7513=ORIENTED_EDGE ( 'NONE', *, *, #6547, .F. ) ;
#7516=EDGE_LOOP ( 'NONE', ( #6879, #2374, #6873, #7539 ) ) ;
#7519=ORIENTED_EDGE ( 'NONE', *, *, #6952, .F. ) ;
#7525=ORIENTED_EDGE ( 'NONE', *, *, #286, .F. ) ;
#7526=VECTOR ( 'NONE', #7753, 1000.000000000000000 ) ;
#7527=DIRECTION ( 'NONE',  ( 0.000000000000000000, 0.000000000000000000, -1.000000000000000000 ) ) ;
#7528=EDGE_CURVE ( 'NONE', #2097, #860, #8079, .T. ) ;
#7538=AXIS2_PLACEMENT_3D ( 'NONE', #7176, #2058, #196 ) ;
#7539=ORIENTED_EDGE ( 'NONE', *, *, #615, .F. ) ;
#7544=CARTESIAN_POINT ( 'NONE',  ( -114.9999999999999147, 115.0000000000000000, 0.000000000000000000 ) ) ;
#7545=DIRECTION ( 'NONE',  ( -1.000000000000000000, 0.000000000000000000, -0.000000000000000000 ) ) ;
#7564=VERTEX_POINT ( 'NONE', #3580 ) ;
#7569=CARTESIAN_POINT ( 'NONE',  ( 14.30908802125418511, 4.500000000000000000, -120.5000000000000284 ) ) ;
#7573=ORIENTED_EDGE ( 'NONE', *, *, #1938, .F. ) ;
#7574=ORIENTED_EDGE ( 'NONE', *, *, #4058, .T. ) ;
#7576=PRODUCT_DEFINITION ( 'UNKNOWN', '', #3260, #2532 ) ;
#7580=CARTESIAN_POINT ( 'NONE',  ( -125.0000000000000000, -120.0000000000000000, 0.000000000000000000 ) ) ;
#7581=EDGE_CURVE ( 'NONE', #2291, #3867, #4901, .T. ) ;
#7585=VERTEX_POINT ( 'NONE', #6043 ) ;
#7587=DIRECTION ( 'NONE',  ( -0.000000000000000000, -0.000000000000000000, -1.000000000000000000 ) ) ;
#7588=DIRECTION ( 'NONE',  ( -0.000000000000000000, 0.000000000000000000, 1.000000000000000000 ) ) ;
#7594=CYLINDRICAL_SURFACE ( 'NONE', #6296, 15.00000000000000000 ) ;
#7597=LINE ( 'NONE', #8232, #6858 ) ;
#7599=ORIENTED_EDGE ( 'NONE', *, *, #5261, .T. ) ;
#7602=EDGE_CURVE ( 'NONE', #805, #326, #5922, .T. ) ;
#7608=EDGE_CURVE ( 'NONE', #7187, #2048, #703, .T. ) ;
#7610=DIRECTION ( 'NONE',  ( -0.000000000000000000, 0.000000000000000000, 1.000000000000000000 ) ) ;
#7612=AXIS2_PLACEMENT_3D ( 'NONE', #6893, #6630, #7270 ) ;
#7613=DIRECTION ( 'NONE',  ( 1.000000000000000000, 0.000000000000000000, 0.000000000000000000 ) ) ;
#7618=CARTESIAN_POINT ( 'NONE',  ( -108.9999999999999147, 115.0000000000000000, 8.205133554287239938E-16 ) ) ;
#7628=FACE_BOUND ( 'NONE', #3190, .T. ) ;
#7641=ORIENTED_EDGE ( 'NONE', *, *, #286, .T. ) ;
#7642=LINE ( 'NONE', #1860, #7132 ) ;
#7651=VECTOR ( 'NONE', #4606, 1000.000000000000000 ) ;
#7654=ORIENTED_EDGE ( 'NONE', *, *, #581, .T. ) ;
#7660=DIRECTION ( 'NONE',  ( -1.000000000000000000, 0.000000000000000000, 0.000000000000000000 ) ) ;
#7662=EDGE_CURVE ( 'NONE', #6525, #4158, #4980, .T. ) ;
#7664=CARTESIAN_POINT ( 'NONE',  ( -114.9999999999999147, 115.0000000000000000, -28.00000000000002487 ) ) ;
#7678=AXIS2_PLACEMENT_3D ( 'NONE', #1607, #1052, #974 ) ;
#7701=CYLINDRICAL_SURFACE ( 'NONE', #2440, 5.999999999999991118 ) ;
#7710=DIRECTION ( 'NONE',  ( -0.000000000000000000, -0.000000000000000000, 1.000000000000000000 ) ) ;
#7724=VECTOR ( 'NONE', #6620, 1000.000000000000000 ) ;
#7725=DIRECTION ( 'NONE',  ( 0.000000000000000000, -1.000000000000000000, 0.000000000000000000 ) ) ;
#7730=ORIENTED_EDGE ( 'NONE', *, *, #4881, .T. ) ;
#7731=ORIENTED_EDGE ( 'NONE', *, *, #295, .F. ) ;
#7735=DIRECTION ( 'NONE',  ( -0.000000000000000000, -0.000000000000000000, -1.000000000000000000 ) ) ;
#7743=EDGE_CURVE ( 'NONE', #2048, #6246, #3097, .T. ) ;
#7753=DIRECTION ( 'NONE',  ( 0.000000000000000000, 1.000000000000000000, 0.000000000000000000 ) ) ;
#7759=ORIENTED_EDGE ( 'NONE', *, *, #6765, .T. ) ;
#7761=DIRECTION ( 'NONE',  ( -1.000000000000000000, 0.000000000000000000, 0.000000000000000000 ) ) ;
#7779=DIRECTION ( 'NONE',  ( -0.000000000000000000, -0.000000000000000000, -1.000000000000000000 ) ) ;
#7782=PLANE ( 'NONE',  #3757 ) ;
#7783=ORIENTED_EDGE ( 'NONE', *, *, #8093, .F. ) ;
#7785=CARTESIAN_POINT ( 'NONE',  ( 0.000000000000000000, 0.000000000000000000, -120.5000000000000284 ) ) ;
#7787=CARTESIAN_POINT ( 'NONE',  ( -25.00000000000000000, 0.000000000000000000, -120.5000000000000284 ) ) ;
#7790=CIRCLE ( 'NONE', #4118, 5.000000000000004441 ) ;
#7792=CARTESIAN_POINT ( 'NONE',  ( 125.0000000000000000, -125.0000000000000000, -28.00000000000002487 ) ) ;
#7795=DIRECTION ( 'NONE',  ( 0.000000000000000000, 0.000000000000000000, -1.000000000000000000 ) ) ;
#7798=EDGE_CURVE ( 'NONE', #6076, #1436, #534, .T. ) ;
#7804=DIRECTION ( 'NONE',  ( -1.000000000000000000, 0.000000000000000000, 0.000000000000000000 ) ) ;
#7810=AXIS2_PLACEMENT_3D ( 'NONE', #370, #2947, #1612 ) ;
#7812=ORIENTED_EDGE ( 'NONE', *, *, #308, .F. ) ;
#7826=AXIS2_PLACEMENT_3D ( 'NONE', #5469, #3593, #6128 ) ;
#7840=CARTESIAN_POINT ( 'NONE',  ( -125.0000000000000000, -120.0000000000000000, -28.00000000000002487 ) ) ;
#7843=CARTESIAN_POINT ( 'NONE',  ( 14.30908802125418511, -4.500000000000000000, -28.00000000000002487 ) ) ;
#7846=FACE_BOUND ( 'NONE', #5222, .T. ) ;
#7847=DIRECTION ( 'NONE',  ( -0.000000000000000000, -0.000000000000000000, 1.000000000000000000 ) ) ;
#7849=CARTESIAN_POINT ( 'NONE',  ( 120.9999999999999005, -115.0000000000000000, 0.000000000000000000 ) ) ;
#7867=APPLICATION_CONTEXT ( 'automotive_design' ) ;
#7870=CARTESIAN_POINT ( 'NONE',  ( -125.0000000000000000, -125.0000000000000000, -28.00000000000002487 ) ) ;
#7871=CARTESIAN_POINT ( 'NONE',  ( 17.61817604250836311, -4.500000000000000000, -28.00000000000002487 ) ) ;
#7876=FACE_OUTER_BOUND ( 'NONE', #4074, .T. ) ;
#7878=ORIENTED_EDGE ( 'NONE', *, *, #1868, .T. ) ;
#7894=PRODUCT ( 'Upright servo motor', 'Upright servo motor', '', ( #7511 ) ) ;
#7908=PLANE ( 'NONE',  #175 ) ;
#7912=ORIENTED_EDGE ( 'NONE', *, *, #2616, .F. ) ;
#7918=DIRECTION ( 'NONE',  ( 1.000000000000000000, 0.000000000000000000, -0.000000000000000000 ) ) ;
#7933=VERTEX_POINT ( 'NONE', #5838 ) ;
#7936=VECTOR ( 'NONE', #2772, 1000.000000000000000 ) ;
#7937=ORIENTED_EDGE ( 'NONE', *, *, #4381, .F. ) ;
#7940=AXIS2_PLACEMENT_3D ( 'NONE', #6783, #5570, #1725 ) ;
#7947=AXIS2_PLACEMENT_3D ( 'NONE', #7422, #1554, #352 ) ;
#7952=VERTEX_POINT ( 'NONE', #2369 ) ;
#7958=DIRECTION ( 'NONE',  ( 0.000000000000000000, -0.000000000000000000, -1.000000000000000000 ) ) ;
#7961=PLANE ( 'NONE',  #8313 ) ;
#7965=FACE_OUTER_BOUND ( 'NONE', #672, .T. ) ;
#7968=DIRECTION ( 'NONE',  ( -0.000000000000000000, -0.000000000000000000, 1.000000000000000000 ) ) ;
#7971=CARTESIAN_POINT ( 'NONE',  ( -120.9999999999999005, 115.0000000000000000, 8.205133554287239938E-16 ) ) ;
#7974=CARTESIAN_POINT ( 'NONE',  ( 125.0000000000000000, -125.0000000000000000, -28.00000000000002487 ) ) ;
#7976=LINE ( 'NONE', #6703, #7281 ) ;
#7986=DIRECTION ( 'NONE',  ( 0.000000000000000000, 0.000000000000000000, -1.000000000000000000 ) ) ;
#7990=EDGE_CURVE ( 'NONE', #5309, #2019, #411, .T. ) ;
#7991=ADVANCED_FACE ( 'NONE', ( #6195 ), #455, .F. ) ;
#8008=VECTOR ( 'NONE', #1403, 1000.000000000000000 ) ;
#8016=VECTOR ( 'NONE', #2969, 1000.000000000000000 ) ;
#8021=CARTESIAN_POINT ( 'NONE',  ( 17.61817604250836311, -4.500000000000000000, -128.0000000000000284 ) ) ;
#8024=DIRECTION ( 'NONE',  ( 0.000000000000000000, 0.000000000000000000, 1.000000000000000000 ) ) ;
#8026=VERTEX_POINT ( 'NONE', #2413 ) ;
#8027=ORIENTED_EDGE ( 'NONE', *, *, #4633, .F. ) ;
#8032=ORIENTED_EDGE ( 'NONE', *, *, #3961, .F. ) ;
#8036=EDGE_LOOP ( 'NONE', ( #6974, #2613, #2209, #2119 ) ) ;
#8037=AXIS2_PLACEMENT_3D ( 'NONE', #5600, #7423, #4184 ) ;
#8041=EDGE_LOOP ( 'NONE', ( #3254, #5806, #3201, #4529 ) ) ;
#8045=LINE ( 'NONE', #2809, #6391 ) ;
#8048=VECTOR ( 'NONE', #4394, 1000.000000000000000 ) ;
#8055=VECTOR ( 'NONE', #5181, 1000.000000000000000 ) ;
#8060=LINE ( 'NONE', #4763, #4472 ) ;
#8064=ORIENTED_EDGE ( 'NONE', *, *, #6929, .T. ) ;
#8066=VECTOR ( 'NONE', #5272, 1000.000000000000000 ) ;
#8070=ORIENTED_EDGE ( 'NONE', *, *, #4685, .F. ) ;
#8079=CIRCLE ( 'NONE', #2098, 5.999999999999991118 ) ;
#8093=EDGE_CURVE ( 'NONE', #381, #1826, #8187, .T. ) ;
#8098=VERTEX_POINT ( 'NONE', #3192 ) ;
#8104=PLANE ( 'NONE',  #5931 ) ;
#8110=DIRECTION ( 'NONE',  ( -1.000000000000000000, 0.000000000000000000, 0.000000000000000000 ) ) ;
#8113=ORIENTED_EDGE ( 'NONE', *, *, #7743, .T. ) ;
#8137=ORIENTED_EDGE ( 'NONE', *, *, #973, .T. ) ;
#8141=ORIENTED_EDGE ( 'NONE', *, *, #1135, .T. ) ;
#8142=AXIS2_PLACEMENT_3D ( 'NONE', #159, #7710, #1928 ) ;
#8147=CARTESIAN_POINT ( 'NONE',  ( 125.0000000000000000, 120.0000000000000000, -28.00000000000002487 ) ) ;
#8153=CARTESIAN_POINT ( 'NONE',  ( -114.9999999999999147, -100.0000000000000000, 250.0000000000000000 ) ) ;
#8160=ORIENTED_EDGE ( 'NONE', *, *, #570, .F. ) ;
#8161=CARTESIAN_POINT ( 'NONE',  ( -120.9999999999999005, 115.0000000000000000, 0.000000000000000000 ) ) ;
#8163=FACE_BOUND ( 'NONE', #1859, .T. ) ;
#8166=ORIENTED_EDGE ( 'NONE', *, *, #3635, .F. ) ;
#8171=ORIENTED_EDGE ( 'NONE', *, *, #190, .F. ) ;
#8173=FACE_OUTER_BOUND ( 'NONE', #8036, .T. ) ;
#8179=PLANE ( 'NONE',  #5769 ) ;
#8183=ORIENTED_EDGE ( 'NONE', *, *, #6434, .T. ) ;
#8187=LINE ( 'NONE', #548, #4714 ) ;
#8188=AXIS2_PLACEMENT_3D ( 'NONE', #5719, #6421, #7761 ) ;
#8195=VECTOR ( 'NONE', #1937, 1000.000000000000000 ) ;
#8196=ORIENTED_EDGE ( 'NONE', *, *, #1285, .T. ) ;
#8197=ORIENTED_EDGE ( 'NONE', *, *, #5260, .F. ) ;
#8210=EDGE_CURVE ( 'NONE', #1618, #4379, #897, .T. ) ;
#8214=LINE ( 'NONE', #7580, #633 ) ;
#8216=CIRCLE ( 'NONE', #2790, 15.00000000000000000 ) ;
#8222=DIRECTION ( 'NONE',  ( -0.000000000000000000, -0.000000000000000000, -1.000000000000000000 ) ) ;
#8224=CARTESIAN_POINT ( 'NONE',  ( 99.99999999999990052, 115.0000000000000000, 250.0000000000000000 ) ) ;
#8228=DIRECTION ( 'NONE',  ( -0.000000000000000000, -0.000000000000000000, 1.000000000000000000 ) ) ;
#8232=CARTESIAN_POINT ( 'NONE',  ( 15.00000000000000000, 0.000000000000000000, -128.0000000000000284 ) ) ;
#8242=ORIENTED_EDGE ( 'NONE', *, *, #7608, .T. ) ;
#8245=DIRECTION ( 'NONE',  ( -0.000000000000000000, -0.000000000000000000, 1.000000000000000000 ) ) ;
#8259=ADVANCED_FACE ( 'NONE', ( #1291 ), #1258, .T. ) ;
#8275=DIRECTION ( 'NONE',  ( 0.000000000000000000, -1.000000000000000000, 0.000000000000000000 ) ) ;
#8280=EDGE_LOOP ( 'NONE', ( #1230, #4333, #4769, #4153 ) ) ;
#8286=CARTESIAN_POINT ( 'NONE',  ( -114.9999999999999147, 115.0000000000000000, 0.000000000000000000 ) ) ;
#8291=AXIS2_PLACEMENT_3D ( 'NONE', #7057, #1278, #3844 ) ;
#8293=LINE ( 'NONE', #5114, #4257 ) ;
#8313=AXIS2_PLACEMENT_3D ( 'NONE', #2192, #5464, #4095 ) ;
#8331=CIRCLE ( 'NONE', #1720, 5.999999999999991118 ) ;
#8332=DIRECTION ( 'NONE',  ( -0.000000000000000000, -0.000000000000000000, -1.000000000000000000 ) ) ;
#8334=DIRECTION ( 'NONE',  ( 1.000000000000000000, 0.000000000000000000, 0.000000000000000000 ) ) ;
#8338=CIRCLE ( 'NONE', #4679, 5.000000000000004441 ) ;
#8344=CARTESIAN_POINT ( 'NONE',  ( -125.0000000000000000, 120.0000000000000000, -28.00000000000002487 ) ) ;
#8387=COLOUR_RGB('Sky Blue',0.24,0.69,0.87);
#8388=FILL_AREA_STYLE_COLOUR('',#8387);
#8389=FILL_AREA_STYLE('',(#8388));
#8390=SURFACE_STYLE_FILL_AREA(#8389);
#8391=SURFACE_SIDE_STYLE('',(#8390));
#8392=SURFACE_STYLE_USAGE(.BOTH.,#8391);
#8393=PRESENTATION_STYLE_ASSIGNMENT((#8392));
ENDSEC;
END-ISO-10303-21;
